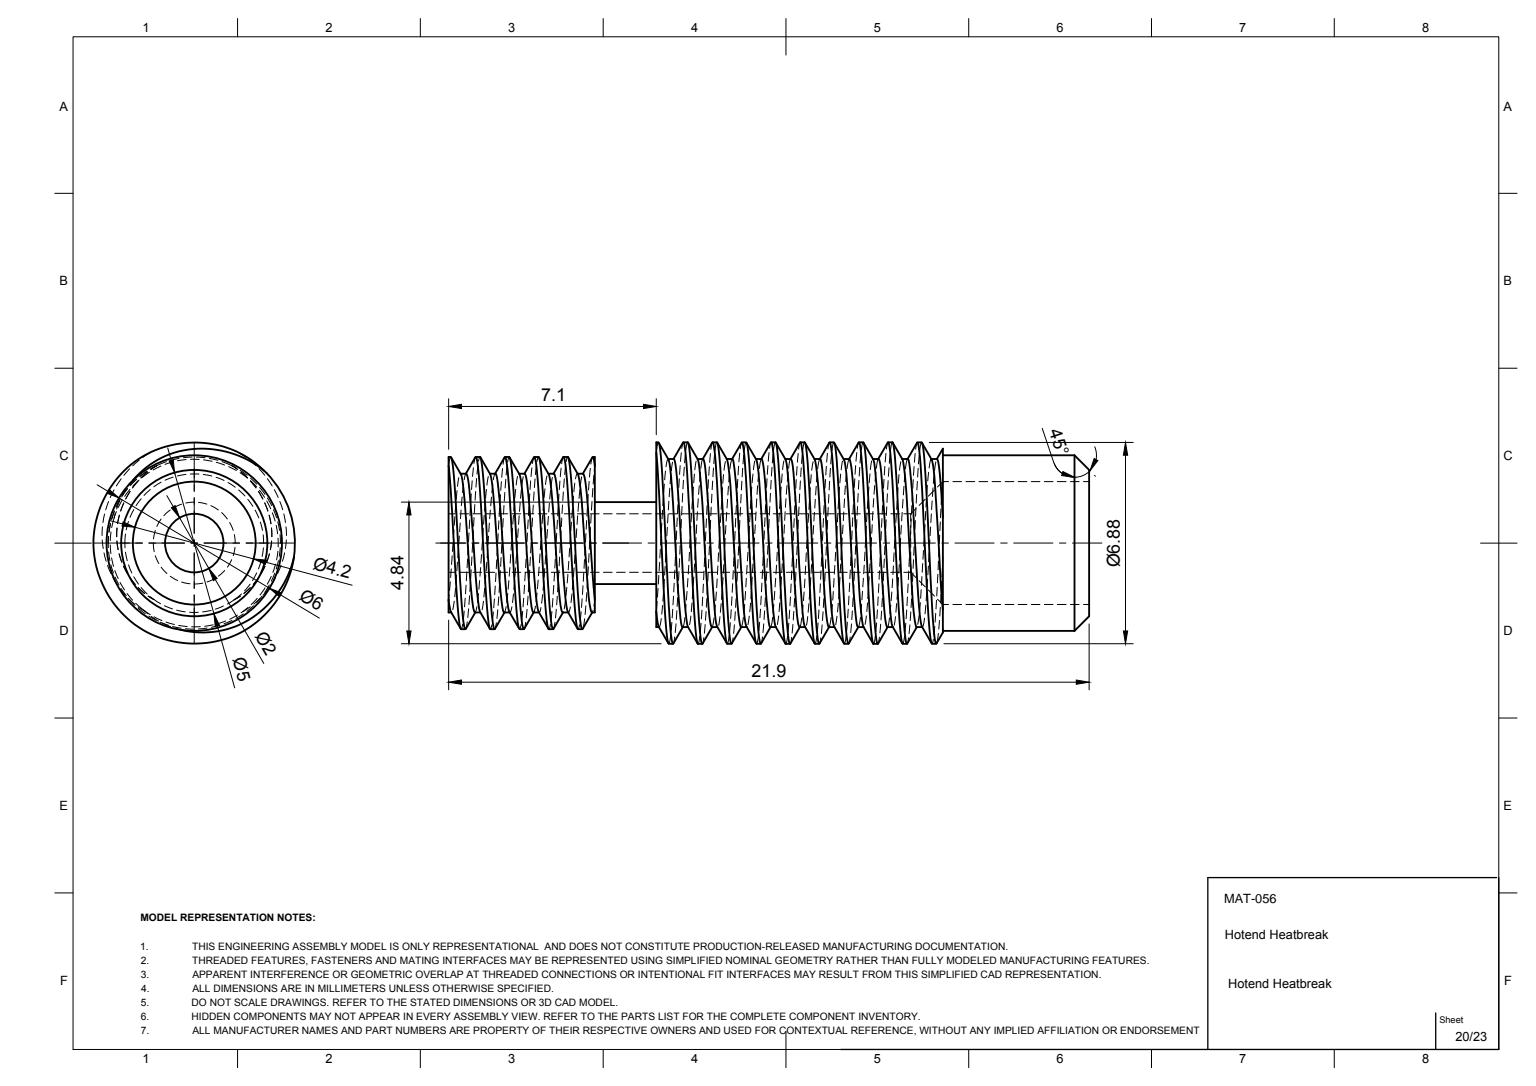
ISO-10303-21;
HEADER;
/* Generated by software containing ST-Developer
 * from STEP Tools, Inc. (www.steptools.com) 
 */

FILE_DESCRIPTION(
/* description */ (''),
/* implementation_level */ '2;1');

FILE_NAME(
/* name */ 'Hotend Heatbreak.step',
/* time_stamp */ '2026-10-28T16:47:13+01:00',
/* author */ (''),
/* organization */ (''),
/* preprocessor_version */ 'ST-DEVELOPER v20.2',
/* originating_system */ 'Autodesk Translation Framework v15.17.0.0',
/* authorisation */ '');

FILE_SCHEMA (('AUTOMOTIVE_DESIGN { 1 0 10303 214 3 1 1 }'));
ENDSEC;

DATA;
#10=MECHANICAL_DESIGN_GEOMETRIC_PRESENTATION_REPRESENTATION('',(#4610),#459242);
#4422=SHAPE_REPRESENTATION_RELATIONSHIP('SRR','None',#459349,#4443);
#4443=ADVANCED_BREP_SHAPE_REPRESENTATION('',(#4490),#459238);
#4490=MANIFOLD_SOLID_BREP('E3D V6 throat',#94668);
#4610=STYLED_ITEM('',(#459519),#4490);
#5107=CONICAL_SURFACE('',#105410,2.5,0.78539816339745);
#5108=CONICAL_SURFACE('',#105423,2.1,0.78539816339745);
#5260=FACE_BOUND('',#18019,.T.);
#5261=FACE_BOUND('',#18033,.T.);
#5262=FACE_BOUND('',#18036,.T.);
#5263=FACE_BOUND('',#18038,.T.);
#6128=PLANE('',#105401);
#6129=PLANE('',#105405);
#6130=PLANE('',#105427);
#6131=PLANE('',#105428);
#6132=PLANE('',#105429);
#6133=PLANE('',#105430);
#6345=B_SPLINE_SURFACE_WITH_KNOTS('',3,3,((#456005,#456006,#456007,#456008,
#456009,#456010,#456011,#456012,#456013,#456014,#456015,#456016,#456017,
#456018,#456019,#456020,#456021,#456022,#456023,#456024,#456025,#456026,
#456027,#456028,#456029,#456030,#456031,#456032,#456033,#456034,#456035,
#456036,#456037,#456038,#456039,#456040,#456041),(#456042,#456043,#456044,
#456045,#456046,#456047,#456048,#456049,#456050,#456051,#456052,#456053,
#456054,#456055,#456056,#456057,#456058,#456059,#456060,#456061,#456062,
#456063,#456064,#456065,#456066,#456067,#456068,#456069,#456070,#456071,
#456072,#456073,#456074,#456075,#456076,#456077,#456078),(#456079,#456080,
#456081,#456082,#456083,#456084,#456085,#456086,#456087,#456088,#456089,
#456090,#456091,#456092,#456093,#456094,#456095,#456096,#456097,#456098,
#456099,#456100,#456101,#456102,#456103,#456104,#456105,#456106,#456107,
#456108,#456109,#456110,#456111,#456112,#456113,#456114,#456115),(#456116,
#456117,#456118,#456119,#456120,#456121,#456122,#456123,#456124,#456125,
#456126,#456127,#456128,#456129,#456130,#456131,#456132,#456133,#456134,
#456135,#456136,#456137,#456138,#456139,#456140,#456141,#456142,#456143,
#456144,#456145,#456146,#456147,#456148,#456149,#456150,#456151,#456152)),
 .UNSPECIFIED.,.F.,.F.,.F.,(4,4),(4,1,1,1,1,1,1,1,1,1,1,1,1,1,1,1,1,1,1,
1,1,1,1,1,1,1,1,1,1,1,1,1,1,1,4),(0.,0.0658467982010768),(8.3074775524011,
9.29231769095425,10.2771578295074,11.2619979680605,12.2468381066137,13.2316782451668,
14.21651838372,15.2013585222731,16.1861986608263,17.1710387993794,18.1558789379326,
19.1407190764857,20.1255592150389,21.110399353592,22.0952394921452,23.0800796306983,
24.0649197692515,25.0497599078046,26.0346000463578,27.0194401849109,28.0042803234641,
28.9891204620172,29.9739606005704,30.9588007391235,31.9436408776767,32.9284810162298,
33.913321154783,34.8981612933361,35.8830014318893,36.8678415704424,37.8526817089956,
38.8375218475487,39.8223619861019,40.807202124655,41.7920422632082),
 .UNSPECIFIED.);
#6346=B_SPLINE_SURFACE_WITH_KNOTS('',3,3,((#456376,#456377,#456378,#456379,
#456380,#456381,#456382,#456383,#456384,#456385,#456386,#456387,#456388,
#456389,#456390,#456391,#456392,#456393,#456394,#456395,#456396,#456397,
#456398,#456399,#456400,#456401,#456402,#456403,#456404,#456405,#456406,
#456407,#456408,#456409,#456410,#456411,#456412),(#456413,#456414,#456415,
#456416,#456417,#456418,#456419,#456420,#456421,#456422,#456423,#456424,
#456425,#456426,#456427,#456428,#456429,#456430,#456431,#456432,#456433,
#456434,#456435,#456436,#456437,#456438,#456439,#456440,#456441,#456442,
#456443,#456444,#456445,#456446,#456447,#456448,#456449),(#456450,#456451,
#456452,#456453,#456454,#456455,#456456,#456457,#456458,#456459,#456460,
#456461,#456462,#456463,#456464,#456465,#456466,#456467,#456468,#456469,
#456470,#456471,#456472,#456473,#456474,#456475,#456476,#456477,#456478,
#456479,#456480,#456481,#456482,#456483,#456484,#456485,#456486),(#456487,
#456488,#456489,#456490,#456491,#456492,#456493,#456494,#456495,#456496,
#456497,#456498,#456499,#456500,#456501,#456502,#456503,#456504,#456505,
#456506,#456507,#456508,#456509,#456510,#456511,#456512,#456513,#456514,
#456515,#456516,#456517,#456518,#456519,#456520,#456521,#456522,#456523)),
 .UNSPECIFIED.,.F.,.F.,.F.,(4,4),(4,1,1,1,1,1,1,1,1,1,1,1,1,1,1,1,1,1,1,
1,1,1,1,1,1,1,1,1,1,1,1,1,1,1,4),(0.,0.0658467982010768),(11.6150328478183,
12.5998729863715,13.5847131249246,14.5695532634778,15.5543934020309,16.5392335405841,
17.5240736791372,18.5089138176904,19.4937539562435,20.4785940947967,21.4634342333498,
22.448274371903,23.4331145104561,24.4179546490093,25.4027947875624,26.3876349261156,
27.3724750646687,28.3573152032219,29.342155341775,30.3269954803282,31.3118356188813,
32.2966757574344,33.2815158959876,34.2663560345407,35.2511961730939,36.236036311647,
37.2208764502002,38.2057165887533,39.1905567273065,40.1753968658596,41.1602370044128,
42.1450771429659,43.1299172815191,44.1147574200722,45.0995975586254),
 .UNSPECIFIED.);
#6347=B_SPLINE_SURFACE_WITH_KNOTS('',3,3,((#456775,#456776,#456777,#456778,
#456779,#456780,#456781,#456782,#456783,#456784,#456785,#456786,#456787,
#456788,#456789,#456790,#456791,#456792,#456793,#456794,#456795,#456796,
#456797,#456798,#456799,#456800,#456801,#456802,#456803,#456804,#456805,
#456806,#456807,#456808,#456809,#456810,#456811,#456812,#456813,#456814,
#456815,#456816,#456817,#456818,#456819,#456820,#456821,#456822,#456823,
#456824,#456825,#456826,#456827,#456828,#456829,#456830,#456831,#456832,
#456833,#456834,#456835,#456836,#456837,#456838,#456839,#456840,#456841),
(#456842,#456843,#456844,#456845,#456846,#456847,#456848,#456849,#456850,
#456851,#456852,#456853,#456854,#456855,#456856,#456857,#456858,#456859,
#456860,#456861,#456862,#456863,#456864,#456865,#456866,#456867,#456868,
#456869,#456870,#456871,#456872,#456873,#456874,#456875,#456876,#456877,
#456878,#456879,#456880,#456881,#456882,#456883,#456884,#456885,#456886,
#456887,#456888,#456889,#456890,#456891,#456892,#456893,#456894,#456895,
#456896,#456897,#456898,#456899,#456900,#456901,#456902,#456903,#456904,
#456905,#456906,#456907,#456908),(#456909,#456910,#456911,#456912,#456913,
#456914,#456915,#456916,#456917,#456918,#456919,#456920,#456921,#456922,
#456923,#456924,#456925,#456926,#456927,#456928,#456929,#456930,#456931,
#456932,#456933,#456934,#456935,#456936,#456937,#456938,#456939,#456940,
#456941,#456942,#456943,#456944,#456945,#456946,#456947,#456948,#456949,
#456950,#456951,#456952,#456953,#456954,#456955,#456956,#456957,#456958,
#456959,#456960,#456961,#456962,#456963,#456964,#456965,#456966,#456967,
#456968,#456969,#456970,#456971,#456972,#456973,#456974,#456975),(#456976,
#456977,#456978,#456979,#456980,#456981,#456982,#456983,#456984,#456985,
#456986,#456987,#456988,#456989,#456990,#456991,#456992,#456993,#456994,
#456995,#456996,#456997,#456998,#456999,#457000,#457001,#457002,#457003,
#457004,#457005,#457006,#457007,#457008,#457009,#457010,#457011,#457012,
#457013,#457014,#457015,#457016,#457017,#457018,#457019,#457020,#457021,
#457022,#457023,#457024,#457025,#457026,#457027,#457028,#457029,#457030,
#457031,#457032,#457033,#457034,#457035,#457036,#457037,#457038,#457039,
#457040,#457041,#457042)),.UNSPECIFIED.,.F.,.F.,.F.,(4,4),(4,1,1,1,1,1,
1,1,1,1,1,1,1,1,1,1,1,1,1,1,1,1,1,1,1,1,1,1,1,1,1,1,1,1,1,1,1,1,1,1,1,1,
1,1,1,1,1,1,1,1,1,1,1,1,1,1,1,1,1,1,1,1,1,1,4),(0.,0.0658179306876173),
(8.30838445208317,9.30280550342046,10.2972265547578,11.2916476060951,12.2860686574324,
13.2804897087697,14.2749107601069,15.2693318114442,16.2637528627815,17.2581739141188,
18.2525949654561,19.2470160167934,20.2414370681307,21.235858119468,22.2302791708053,
23.2247002221426,24.2191212734799,25.2135423248172,26.2079633761545,27.2023844274918,
28.1968054788291,29.1912265301664,30.1856475815037,31.180068632841,32.1744896841783,
33.1689107355156,34.1633317868529,35.1577528381902,36.1521738895275,37.1465949408648,
38.1410159922021,39.1354370435394,40.1298580948767,41.1242791462139,42.1187001975512,
43.1131212488885,44.1075423002258,45.1019633515631,46.0963844029004,47.0908054542377,
48.085226505575,49.0796475569123,50.0740686082496,51.0684896595869,52.0629107109242,
53.0573317622615,54.0517528135988,55.0461738649361,56.0405949162734,57.0350159676107,
58.029437018948,59.0238580702853,60.0182791216226,61.0127001729599,62.0071212242972,
63.0015422756345,63.9959633269718,64.9903843783091,65.9848054296463,66.9792264809836,
67.9736475323209,68.9680685836582,69.9624896349955,70.9569106863328,71.9513317376701),
 .UNSPECIFIED.);
#6348=B_SPLINE_SURFACE_WITH_KNOTS('',3,3,((#457239,#457240,#457241,#457242,
#457243,#457244,#457245,#457246,#457247,#457248,#457249,#457250,#457251,
#457252,#457253,#457254,#457255,#457256,#457257,#457258,#457259,#457260,
#457261,#457262,#457263,#457264,#457265,#457266,#457267,#457268,#457269,
#457270,#457271,#457272,#457273,#457274,#457275,#457276,#457277,#457278,
#457279,#457280,#457281,#457282,#457283,#457284,#457285,#457286,#457287,
#457288,#457289,#457290,#457291,#457292,#457293,#457294,#457295,#457296,
#457297,#457298,#457299,#457300,#457301,#457302,#457303,#457304,#457305),
(#457306,#457307,#457308,#457309,#457310,#457311,#457312,#457313,#457314,
#457315,#457316,#457317,#457318,#457319,#457320,#457321,#457322,#457323,
#457324,#457325,#457326,#457327,#457328,#457329,#457330,#457331,#457332,
#457333,#457334,#457335,#457336,#457337,#457338,#457339,#457340,#457341,
#457342,#457343,#457344,#457345,#457346,#457347,#457348,#457349,#457350,
#457351,#457352,#457353,#457354,#457355,#457356,#457357,#457358,#457359,
#457360,#457361,#457362,#457363,#457364,#457365,#457366,#457367,#457368,
#457369,#457370,#457371,#457372),(#457373,#457374,#457375,#457376,#457377,
#457378,#457379,#457380,#457381,#457382,#457383,#457384,#457385,#457386,
#457387,#457388,#457389,#457390,#457391,#457392,#457393,#457394,#457395,
#457396,#457397,#457398,#457399,#457400,#457401,#457402,#457403,#457404,
#457405,#457406,#457407,#457408,#457409,#457410,#457411,#457412,#457413,
#457414,#457415,#457416,#457417,#457418,#457419,#457420,#457421,#457422,
#457423,#457424,#457425,#457426,#457427,#457428,#457429,#457430,#457431,
#457432,#457433,#457434,#457435,#457436,#457437,#457438,#457439),(#457440,
#457441,#457442,#457443,#457444,#457445,#457446,#457447,#457448,#457449,
#457450,#457451,#457452,#457453,#457454,#457455,#457456,#457457,#457458,
#457459,#457460,#457461,#457462,#457463,#457464,#457465,#457466,#457467,
#457468,#457469,#457470,#457471,#457472,#457473,#457474,#457475,#457476,
#457477,#457478,#457479,#457480,#457481,#457482,#457483,#457484,#457485,
#457486,#457487,#457488,#457489,#457490,#457491,#457492,#457493,#457494,
#457495,#457496,#457497,#457498,#457499,#457500,#457501,#457502,#457503,
#457504,#457505,#457506)),.UNSPECIFIED.,.F.,.F.,.F.,(4,4),(4,1,1,1,1,1,
1,1,1,1,1,1,1,1,1,1,1,1,1,1,1,1,1,1,1,1,1,1,1,1,1,1,1,1,1,1,1,1,1,1,1,1,
1,1,1,1,1,1,1,1,1,1,1,1,1,1,1,1,1,1,1,1,1,1,4),(0.,0.0658179306876173),
(11.6150328478183,12.6094538991556,13.6038749504929,14.5982960018302,15.5927170531675,
16.5871381045047,17.581559155842,18.5759802071793,19.5704012585166,20.5648223098539,
21.5592433611912,22.5536644125285,23.5480854638658,24.5425065152031,25.5369275665404,
26.5313486178777,27.525769669215,28.5201907205523,29.5146117718896,30.5090328232269,
31.5034538745642,32.4978749259015,33.4922959772388,34.4867170285761,35.4811380799134,
36.4755591312507,37.469980182588,38.4644012339253,39.4588222852626,40.4532433365999,
41.4476643879372,42.4420854392745,43.4365064906117,44.430927541949,45.4253485932863,
46.4197696446236,47.4141906959609,48.4086117472982,49.4030327986355,50.3974538499728,
51.3918749013101,52.3862959526474,53.3807170039847,54.375138055322,55.3695591066593,
56.3639801579966,57.3584012093339,58.3528222606712,59.3472433120085,60.3416643633458,
61.3360854146831,62.3305064660204,63.3249275173577,64.319348568695,65.3137696200323,
66.3081906713696,67.3026117227069,68.2970327740442,69.2914538253815,70.2858748767188,
71.280295928056,72.2747169793933,73.2691380307306,74.2635590820679,75.2579801334052),
 .UNSPECIFIED.);
#12030=FACE_OUTER_BOUND('',#17985,.T.);
#12031=FACE_OUTER_BOUND('',#17986,.T.);
#12032=FACE_OUTER_BOUND('',#17987,.T.);
#12033=FACE_OUTER_BOUND('',#17988,.T.);
#12034=FACE_OUTER_BOUND('',#17989,.T.);
#12035=FACE_OUTER_BOUND('',#17990,.T.);
#12036=FACE_OUTER_BOUND('',#17991,.T.);
#12037=FACE_OUTER_BOUND('',#17992,.T.);
#12038=FACE_OUTER_BOUND('',#17993,.T.);
#12039=FACE_OUTER_BOUND('',#17994,.T.);
#12040=FACE_OUTER_BOUND('',#17995,.T.);
#12041=FACE_OUTER_BOUND('',#17996,.T.);
#12042=FACE_OUTER_BOUND('',#17997,.T.);
#12043=FACE_OUTER_BOUND('',#17998,.T.);
#12044=FACE_OUTER_BOUND('',#17999,.T.);
#12045=FACE_OUTER_BOUND('',#18000,.T.);
#12046=FACE_OUTER_BOUND('',#18001,.T.);
#12047=FACE_OUTER_BOUND('',#18002,.T.);
#12048=FACE_OUTER_BOUND('',#18003,.T.);
#12049=FACE_OUTER_BOUND('',#18004,.T.);
#12050=FACE_OUTER_BOUND('',#18005,.T.);
#12051=FACE_OUTER_BOUND('',#18006,.T.);
#12052=FACE_OUTER_BOUND('',#18007,.T.);
#12053=FACE_OUTER_BOUND('',#18008,.T.);
#12054=FACE_OUTER_BOUND('',#18009,.T.);
#12055=FACE_OUTER_BOUND('',#18010,.T.);
#12056=FACE_OUTER_BOUND('',#18011,.T.);
#12057=FACE_OUTER_BOUND('',#18012,.T.);
#12058=FACE_OUTER_BOUND('',#18013,.T.);
#12059=FACE_OUTER_BOUND('',#18014,.T.);
#12060=FACE_OUTER_BOUND('',#18015,.T.);
#12061=FACE_OUTER_BOUND('',#18016,.T.);
#12062=FACE_OUTER_BOUND('',#18017,.T.);
#12063=FACE_OUTER_BOUND('',#18018,.T.);
#12064=FACE_OUTER_BOUND('',#18020,.T.);
#12065=FACE_OUTER_BOUND('',#18021,.T.);
#12066=FACE_OUTER_BOUND('',#18022,.T.);
#12067=FACE_OUTER_BOUND('',#18023,.T.);
#12068=FACE_OUTER_BOUND('',#18024,.T.);
#12069=FACE_OUTER_BOUND('',#18025,.T.);
#12070=FACE_OUTER_BOUND('',#18026,.T.);
#12071=FACE_OUTER_BOUND('',#18027,.T.);
#12072=FACE_OUTER_BOUND('',#18028,.T.);
#12073=FACE_OUTER_BOUND('',#18029,.T.);
#12074=FACE_OUTER_BOUND('',#18030,.T.);
#12075=FACE_OUTER_BOUND('',#18031,.T.);
#12076=FACE_OUTER_BOUND('',#18032,.T.);
#12077=FACE_OUTER_BOUND('',#18034,.T.);
#12078=FACE_OUTER_BOUND('',#18035,.T.);
#12079=FACE_OUTER_BOUND('',#18037,.T.);
#17985=EDGE_LOOP('',(#86428,#86429,#86430,#86431));
#17986=EDGE_LOOP('',(#86432,#86433,#86434,#86435));
#17987=EDGE_LOOP('',(#86436,#86437,#86438,#86439));
#17988=EDGE_LOOP('',(#86440,#86441,#86442,#86443));
#17989=EDGE_LOOP('',(#86444,#86445,#86446,#86447));
#17990=EDGE_LOOP('',(#86448,#86449,#86450,#86451));
#17991=EDGE_LOOP('',(#86452,#86453,#86454,#86455));
#17992=EDGE_LOOP('',(#86456,#86457,#86458,#86459));
#17993=EDGE_LOOP('',(#86460,#86461,#86462,#86463));
#17994=EDGE_LOOP('',(#86464,#86465,#86466,#86467));
#17995=EDGE_LOOP('',(#86468,#86469,#86470));
#17996=EDGE_LOOP('',(#86471,#86472,#86473,#86474,#86475));
#17997=EDGE_LOOP('',(#86476,#86477,#86478,#86479));
#17998=EDGE_LOOP('',(#86480,#86481,#86482,#86483));
#17999=EDGE_LOOP('',(#86484,#86485,#86486,#86487));
#18000=EDGE_LOOP('',(#86488,#86489,#86490,#86491));
#18001=EDGE_LOOP('',(#86492,#86493,#86494,#86495));
#18002=EDGE_LOOP('',(#86496,#86497,#86498,#86499));
#18003=EDGE_LOOP('',(#86500,#86501,#86502,#86503));
#18004=EDGE_LOOP('',(#86504,#86505,#86506,#86507));
#18005=EDGE_LOOP('',(#86508,#86509,#86510,#86511));
#18006=EDGE_LOOP('',(#86512,#86513,#86514,#86515));
#18007=EDGE_LOOP('',(#86516,#86517,#86518,#86519));
#18008=EDGE_LOOP('',(#86520,#86521,#86522,#86523));
#18009=EDGE_LOOP('',(#86524,#86525,#86526,#86527));
#18010=EDGE_LOOP('',(#86528,#86529,#86530,#86531));
#18011=EDGE_LOOP('',(#86532,#86533,#86534,#86535));
#18012=EDGE_LOOP('',(#86536,#86537,#86538,#86539));
#18013=EDGE_LOOP('',(#86540,#86541,#86542,#86543));
#18014=EDGE_LOOP('',(#86544,#86545,#86546,#86547));
#18015=EDGE_LOOP('',(#86548,#86549,#86550,#86551,#86552,#86553,#86554,#86555,
#86556,#86557,#86558,#86559,#86560,#86561));
#18016=EDGE_LOOP('',(#86562,#86563,#86564,#86565));
#18017=EDGE_LOOP('',(#86566,#86567,#86568,#86569,#86570,#86571,#86572,#86573,
#86574,#86575,#86576,#86577,#86578,#86579));
#18018=EDGE_LOOP('',(#86580,#86581,#86582,#86583));
#18019=EDGE_LOOP('',(#86584));
#18020=EDGE_LOOP('',(#86585,#86586,#86587,#86588));
#18021=EDGE_LOOP('',(#86589,#86590,#86591,#86592,#86593,#86594));
#18022=EDGE_LOOP('',(#86595,#86596,#86597,#86598,#86599,#86600,#86601,#86602,
#86603,#86604,#86605,#86606,#86607,#86608,#86609,#86610,#86611,#86612,#86613,
#86614,#86615,#86616,#86617,#86618));
#18023=EDGE_LOOP('',(#86619,#86620,#86621,#86622));
#18024=EDGE_LOOP('',(#86623,#86624,#86625,#86626,#86627,#86628,#86629,#86630,
#86631,#86632,#86633,#86634,#86635,#86636,#86637,#86638,#86639,#86640,#86641,
#86642,#86643,#86644,#86645,#86646,#86647));
#18025=EDGE_LOOP('',(#86648,#86649,#86650,#86651,#86652));
#18026=EDGE_LOOP('',(#86653,#86654,#86655,#86656));
#18027=EDGE_LOOP('',(#86657,#86658,#86659,#86660));
#18028=EDGE_LOOP('',(#86661,#86662,#86663,#86664,#86665,#86666,#86667));
#18029=EDGE_LOOP('',(#86668,#86669,#86670,#86671));
#18030=EDGE_LOOP('',(#86672,#86673,#86674,#86675));
#18031=EDGE_LOOP('',(#86676,#86677,#86678,#86679));
#18032=EDGE_LOOP('',(#86680));
#18033=EDGE_LOOP('',(#86681));
#18034=EDGE_LOOP('',(#86682,#86683,#86684,#86685));
#18035=EDGE_LOOP('',(#86686,#86687,#86688,#86689));
#18036=EDGE_LOOP('',(#86690));
#18037=EDGE_LOOP('',(#86691,#86692,#86693,#86694));
#18038=EDGE_LOOP('',(#86695));
#23442=CIRCLE('',#105365,3.442);
#23443=CIRCLE('',#105376,2.872);
#23444=CIRCLE('',#105378,2.872);
#23445=CIRCLE('',#105388,2.942);
#23446=CIRCLE('',#105394,2.37175);
#23447=CIRCLE('',#105400,2.37175);
#23448=CIRCLE('',#105402,2.942);
#23449=CIRCLE('',#105403,1.4);
#23450=CIRCLE('',#105406,3.);
#23451=CIRCLE('',#105407,3.);
#23452=CIRCLE('',#105409,2.872);
#23453=CIRCLE('',#105411,3.);
#23454=CIRCLE('',#105412,3.);
#23455=CIRCLE('',#105413,2.5);
#23456=CIRCLE('',#105415,1.4);
#23457=CIRCLE('',#105417,3.442);
#23458=CIRCLE('',#105419,3.);
#23459=CIRCLE('',#105421,2.1);
#23460=CIRCLE('',#105422,2.1);
#23461=CIRCLE('',#105424,1.);
#23462=CIRCLE('',#105426,1.);
#26936=B_SPLINE_CURVE_WITH_KNOTS('',3,(#454971,#454972,#454973,#454974,
#454975,#454976,#454977,#454978,#454979,#454980),.UNSPECIFIED.,.F.,.F.,
(4,3,3,4),(-4.09293042013066,-3.97768420534918,-2.98326315401189,-2.06773127522702),
 .UNSPECIFIED.);
#26937=B_SPLINE_CURVE_WITH_KNOTS('',3,(#454983,#454984,#454985,#454986,
#454987,#454988,#454989),.UNSPECIFIED.,.F.,.F.,(4,3,4),(0.,0.994421051337293,
1.11639350868612),.UNSPECIFIED.);
#26938=B_SPLINE_CURVE_WITH_KNOTS('',3,(#454994,#454995,#454996,#454997,
#454998,#454999,#455000,#455001,#455002,#455003,#455004,#455005,#455006,
#455007,#455008,#455009,#455010,#455011,#455012,#455013,#455014,#455015),
 .UNSPECIFIED.,.F.,.F.,(4,3,3,3,3,3,3,4),(-10.3761157273102,-9.94421051337296,
-8.94978946203567,-7.95536841069837,-6.96094735936108,-5.96652630802378,
-4.97210525668648,-4.09293042013066),.UNSPECIFIED.);
#26939=B_SPLINE_CURVE_WITH_KNOTS('',3,(#455016,#455017,#455018,#455019,
#455020,#455021,#455022,#455023,#455024,#455025,#455026,#455027,#455028,
#455029,#455030,#455031,#455032,#455033,#455034,#455035,#455036,#455037),
 .UNSPECIFIED.,.F.,.F.,(4,3,3,3,3,3,3,4),(1.11639350868612,1.98884210267459,
2.98326315401189,3.97768420534918,4.97210525668648,5.96652630802378,6.96094735936107,
7.39957881586571),.UNSPECIFIED.);
#26940=B_SPLINE_CURVE_WITH_KNOTS('',3,(#455042,#455043,#455044,#455045,
#455046,#455047,#455048,#455049,#455050,#455051,#455052,#455053,#455054,
#455055,#455056,#455057,#455058,#455059,#455060,#455061,#455062,#455063),
 .UNSPECIFIED.,.F.,.F.,(4,3,3,3,3,3,3,4),(-16.6593010344898,-15.9107368213967,
-14.9163157700594,-13.9218947187222,-12.9274736673849,-11.9330526160476,
-10.9386315647103,-10.3761157273102),.UNSPECIFIED.);
#26941=B_SPLINE_CURVE_WITH_KNOTS('',3,(#455064,#455065,#455066,#455067,
#455068,#455069,#455070,#455071,#455072,#455073,#455074,#455075,#455076,
#455077,#455078,#455079,#455080,#455081,#455082,#455083,#455084,#455085),
 .UNSPECIFIED.,.F.,.F.,(4,3,3,3,3,3,3,4),(7.39957881586571,7.95536841069837,
8.94978946203567,9.94421051337297,10.9386315647103,11.9330526160476,12.9274736673849,
13.6827641230453),.UNSPECIFIED.);
#26942=B_SPLINE_CURVE_WITH_KNOTS('',3,(#455090,#455091,#455092,#455093,
#455094,#455095,#455096,#455097,#455098,#455099,#455100,#455101,#455102,
#455103,#455104,#455105,#455106,#455107,#455108,#455109,#455110,#455111,
#455112,#455113,#455114),.UNSPECIFIED.,.F.,.F.,(4,3,3,3,3,3,3,3,4),(-22.9424863416694,
-22.8716841807578,-21.8772631294205,-20.8828420780832,-19.8884210267459,
-18.8939999754086,-17.8995789240713,-16.905157872734,-16.6593010344898),
 .UNSPECIFIED.);
#26943=B_SPLINE_CURVE_WITH_KNOTS('',3,(#455115,#455116,#455117,#455118,
#455119,#455120,#455121,#455122,#455123,#455124,#455125,#455126,#455127,
#455128,#455129,#455130,#455131,#455132,#455133,#455134,#455135,#455136,
#455137,#455138,#455139),.UNSPECIFIED.,.F.,.F.,(4,3,3,3,3,3,3,3,4),(13.6827641230453,
13.9218947187222,14.9163157700594,15.9107368213967,16.905157872734,17.8995789240713,
18.8939999754086,19.8884210267459,19.9659494302249),.UNSPECIFIED.);
#26944=B_SPLINE_CURVE_WITH_KNOTS('',3,(#455144,#455145,#455146,#455147,
#455148,#455149,#455150,#455151,#455152,#455153,#455154,#455155,#455156,
#455157,#455158,#455159,#455160,#455161,#455162,#455163,#455164,#455165),
 .UNSPECIFIED.,.F.,.F.,(4,3,3,3,3,3,3,4),(-29.225671648849,-28.8382104887816,
-27.8437894374443,-26.849368386107,-25.8549473347697,-24.8605262834324,
-23.8661052320951,-22.9424863416694),.UNSPECIFIED.);
#26945=B_SPLINE_CURVE_WITH_KNOTS('',3,(#455166,#455167,#455168,#455169,
#455170,#455171,#455172,#455173,#455174,#455175,#455176,#455177,#455178,
#455179,#455180,#455181,#455182,#455183,#455184,#455185,#455186,#455187),
 .UNSPECIFIED.,.F.,.F.,(4,3,3,3,3,3,3,4),(19.9659494302249,20.8828420780832,
21.8772631294205,22.8716841807578,23.8661052320951,24.8605262834324,25.8549473347697,
26.2491347374045),.UNSPECIFIED.);
#26946=B_SPLINE_CURVE_WITH_KNOTS('',3,(#455192,#455193,#455194,#455195,
#455196,#455197,#455198,#455199,#455200,#455201,#455202,#455203,#455204,
#455205,#455206,#455207,#455208,#455209,#455210,#455211,#455212,#455213),
 .UNSPECIFIED.,.F.,.F.,(4,3,3,3,3,3,3,4),(-35.5088569560286,-34.8047367968054,
-33.8103157454681,-32.8158946941308,-31.8214736427935,-30.8270525914562,
-29.8326315401189,-29.225671648849),.UNSPECIFIED.);
#26947=B_SPLINE_CURVE_WITH_KNOTS('',3,(#455214,#455215,#455216,#455217,
#455218,#455219,#455220,#455221,#455222,#455223,#455224,#455225,#455226,
#455227,#455228,#455229,#455230,#455231,#455232,#455233,#455234,#455235),
 .UNSPECIFIED.,.F.,.F.,(4,3,3,3,3,3,3,4),(26.2491347374045,26.849368386107,
27.8437894374443,28.8382104887816,29.8326315401189,30.8270525914562,31.8214736427935,
32.532320044584),.UNSPECIFIED.);
#26948=B_SPLINE_CURVE_WITH_KNOTS('',3,(#455240,#455241,#455242,#455243,
#455244,#455245,#455246,#455247,#455248,#455249,#455250,#455251,#455252,
#455253,#455254,#455255,#455256,#455257,#455258,#455259,#455260,#455261,
#455262,#455263,#455264),.UNSPECIFIED.,.F.,.F.,(4,3,3,3,3,3,3,3,4),(-41.7920422632082,
-41.7656841561665,-40.7712631048292,-39.7768420534919,-38.7824210021546,
-37.7879999508173,-36.79357889948,-35.7991578481427,-35.5088569560286),
 .UNSPECIFIED.);
#26949=B_SPLINE_CURVE_WITH_KNOTS('',3,(#455265,#455266,#455267,#455268,
#455269,#455270,#455271,#455272,#455273,#455274,#455275,#455276,#455277,
#455278,#455279,#455280,#455281,#455282,#455283,#455284,#455285,#455286,
#455287,#455288,#455289),.UNSPECIFIED.,.F.,.F.,(4,3,3,3,3,3,3,3,4),(32.532320044584,
32.8158946941308,33.8103157454681,34.8047367968054,35.7991578481427,36.79357889948,
37.7879999508173,38.7824210021546,38.8155053517636),.UNSPECIFIED.);
#26950=B_SPLINE_CURVE_WITH_KNOTS('',3,(#455294,#455295,#455296,#455297,
#455298,#455299,#455300,#455301,#455302,#455303,#455304,#455305,#455306,
#455307,#455308,#455309,#455310,#455311,#455312,#455313,#455314,#455315),
 .UNSPECIFIED.,.F.,.F.,(4,3,3,3,3,3,3,4),(-48.0752275703878,-47.7322104641902,
-46.7377894128529,-45.7433683615156,-44.7489473101783,-43.754526258841,
-42.7601052075037,-41.7920422632082),.UNSPECIFIED.);
#26951=B_SPLINE_CURVE_WITH_KNOTS('',3,(#455316,#455317,#455318,#455319,
#455320,#455321,#455322,#455323,#455324,#455325,#455326,#455327,#455328,
#455329,#455330,#455331,#455332,#455333,#455334,#455335,#455336,#455337),
 .UNSPECIFIED.,.F.,.F.,(4,3,3,3,3,3,3,4),(38.8155053517636,39.7768420534919,
40.7712631048292,41.7656841561664,42.7601052075037,43.754526258841,44.7489473101783,
45.0986906589432),.UNSPECIFIED.);
#26952=B_SPLINE_CURVE_WITH_KNOTS('',3,(#455342,#455343,#455344,#455345,
#455346,#455347,#455348,#455349,#455350,#455351,#455352,#455353,#455354,
#455355,#455356,#455357,#455358,#455359,#455360,#455361,#455362,#455363),
 .UNSPECIFIED.,.F.,.F.,(4,3,3,3,3,3,3,4),(-54.3584128775674,-53.698736772214,
-52.7043157208767,-51.7098946695394,-50.7154736182021,-49.7210525668648,
-48.7266315155275,-48.0752275703878),.UNSPECIFIED.);
#26953=B_SPLINE_CURVE_WITH_KNOTS('',3,(#455364,#455365,#455366,#455367,
#455368,#455369,#455370,#455371,#455372,#455373,#455374,#455375,#455376,
#455377,#455378,#455379,#455380,#455381,#455382,#455383,#455384,#455385),
 .UNSPECIFIED.,.F.,.F.,(4,3,3,3,3,3,3,4),(45.0986906589432,45.7433683615156,
46.7377894128529,47.7322104641902,48.7266315155275,49.7210525668648,50.7154736182021,
51.3818759661228),.UNSPECIFIED.);
#26954=B_SPLINE_CURVE_WITH_KNOTS('',3,(#455390,#455391,#455392,#455393,
#455394,#455395,#455396,#455397,#455398,#455399,#455400,#455401,#455402,
#455403,#455404,#455405,#455406,#455407,#455408,#455409,#455410,#455411),
 .UNSPECIFIED.,.F.,.F.,(4,3,3,3,3,3,3,4),(-60.641598184747,-59.6652630802378,
-58.6708420289005,-57.6764209775632,-56.6819999262259,-55.6875788748886,
-54.6931578235513,-54.3584128775674),.UNSPECIFIED.);
#26955=B_SPLINE_CURVE_WITH_KNOTS('',3,(#455412,#455413,#455414,#455415,
#455416,#455417,#455418,#455419,#455420,#455421,#455422,#455423,#455424,
#455425,#455426,#455427,#455428,#455429,#455430,#455431,#455432,#455433),
 .UNSPECIFIED.,.F.,.F.,(4,3,3,3,3,3,3,4),(51.3818759661228,51.7098946695394,
52.7043157208767,53.698736772214,54.6931578235513,55.6875788748886,56.6819999262259,
57.6650612733024),.UNSPECIFIED.);
#26956=B_SPLINE_CURVE_WITH_KNOTS('',3,(#455439,#455440,#455441,#455442,
#455443),.UNSPECIFIED.,.F.,.F.,(4,1,4),(72.2566310325653,72.2747169793933,
73.1902488581782),.UNSPECIFIED.);
#26957=B_SPLINE_CURVE_WITH_KNOTS('',3,(#455449,#455450,#455451,#455452,
#455453,#455454,#455455,#455456,#455457,#455458),.UNSPECIFIED.,.F.,.F.,
(4,1,1,1,1,1,1,4),(65.9734457253856,66.3081906713696,67.3026117227069,68.2970327740442,
69.2914538253815,70.2858748767188,71.280295928056,72.2566310325653),
 .UNSPECIFIED.);
#26958=B_SPLINE_CURVE_WITH_KNOTS('',3,(#455461,#455462,#455463,#455464,
#455465,#455466,#455467,#455468,#455469,#455470),.UNSPECIFIED.,.F.,.F.,
(4,1,1,1,1,1,1,4),(65.9734457253856,65.9848054296463,66.9792264809836,67.9736475323209,
68.9680685836582,69.9624896349955,70.9569106863328,71.9513317376701),
 .UNSPECIFIED.);
#26959=B_SPLINE_CURVE_WITH_KNOTS('',3,(#455475,#455476,#455477,#455478,
#455479,#455480,#455481,#455482,#455483,#455484),.UNSPECIFIED.,.F.,.F.,
(4,1,1,1,1,1,1,4),(59.6902604182061,60.3416643633458,61.3360854146831,62.3305064660204,
63.3249275173577,64.319348568695,65.3137696200323,65.9734457253856),
 .UNSPECIFIED.);
#26960=B_SPLINE_CURVE_WITH_KNOTS('',3,(#455485,#455486,#455487,#455488,
#455489,#455490,#455491,#455492,#455493,#455494),.UNSPECIFIED.,.F.,.F.,
(4,1,1,1,1,1,1,4),(59.6902604182061,60.0182791216226,61.0127001729599,62.0071212242972,
63.0015422756345,63.9959633269718,64.9903843783091,65.9734457253856),
 .UNSPECIFIED.);
#26961=B_SPLINE_CURVE_WITH_KNOTS('',3,(#455499,#455500,#455501,#455502,
#455503,#455504,#455505,#455506,#455507,#455508),.UNSPECIFIED.,.F.,.F.,
(4,1,1,1,1,1,1,4),(53.4070751110265,54.375138055322,55.3695591066593,56.3639801579966,
57.3584012093339,58.3528222606712,59.3472433120085,59.6902604182061),
 .UNSPECIFIED.);
#26962=B_SPLINE_CURVE_WITH_KNOTS('',3,(#455509,#455510,#455511,#455512,
#455513,#455514,#455515,#455516,#455517,#455518),.UNSPECIFIED.,.F.,.F.,
(4,1,1,1,1,1,1,4),(53.4070751110265,54.0517528135988,55.0461738649361,56.0405949162734,
57.0350159676107,58.029437018948,59.0238580702853,59.6902604182061),
 .UNSPECIFIED.);
#26963=B_SPLINE_CURVE_WITH_KNOTS('',3,(#455523,#455524,#455525,#455526,
#455527,#455528,#455529,#455530,#455531,#455532,#455533),.UNSPECIFIED.,
 .F.,.F.,(4,1,1,1,1,1,1,1,4),(47.1238898038469,47.4141906959609,48.4086117472982,
49.4030327986355,50.3974538499728,51.3918749013101,52.3862959526474,53.3807170039847,
53.4070751110265),.UNSPECIFIED.);
#26964=B_SPLINE_CURVE_WITH_KNOTS('',3,(#455534,#455535,#455536,#455537,
#455538,#455539,#455540,#455541,#455542,#455543),.UNSPECIFIED.,.F.,.F.,
(4,1,1,1,1,1,1,4),(47.1238898038469,48.085226505575,49.0796475569123,50.0740686082496,
51.0684896595869,52.0629107109242,53.0573317622615,53.4070751110265),
 .UNSPECIFIED.);
#26965=B_SPLINE_CURVE_WITH_KNOTS('',3,(#455548,#455549,#455550,#455551,
#455552,#455553,#455554,#455555,#455556,#455557),.UNSPECIFIED.,.F.,.F.,
(4,1,1,1,1,1,1,4),(40.8407044966673,41.4476643879372,42.4420854392745,43.4365064906117,
44.430927541949,45.4253485932863,46.4197696446236,47.1238898038469),
 .UNSPECIFIED.);
#26966=B_SPLINE_CURVE_WITH_KNOTS('',3,(#455558,#455559,#455560,#455561,
#455562,#455563,#455564,#455565,#455566,#455567,#455568),.UNSPECIFIED.,
 .F.,.F.,(4,1,1,1,1,1,1,1,4),(40.8407044966673,41.1242791462139,42.1187001975512,
43.1131212488885,44.1075423002258,45.1019633515631,46.0963844029004,47.0908054542377,
47.1238898038469),.UNSPECIFIED.);
#26967=B_SPLINE_CURVE_WITH_KNOTS('',3,(#455573,#455574,#455575,#455576,
#455577,#455578,#455579,#455580,#455581,#455582),.UNSPECIFIED.,.F.,.F.,
(4,1,1,1,1,1,1,4),(34.5575191894877,35.4811380799134,36.4755591312507,37.469980182588,
38.4644012339253,39.4588222852626,40.4532433365999,40.8407044966673),
 .UNSPECIFIED.);
#26968=B_SPLINE_CURVE_WITH_KNOTS('',3,(#455583,#455584,#455585,#455586,
#455587,#455588,#455589,#455590,#455591,#455592),.UNSPECIFIED.,.F.,.F.,
(4,1,1,1,1,1,1,4),(34.5575191894877,35.1577528381902,36.1521738895275,37.1465949408648,
38.1410159922021,39.1354370435394,40.1298580948767,40.8407044966673),
 .UNSPECIFIED.);
#26969=B_SPLINE_CURVE_WITH_KNOTS('',3,(#455597,#455598,#455599,#455600,
#455601,#455602,#455603,#455604,#455605,#455606,#455607),.UNSPECIFIED.,
 .F.,.F.,(4,1,1,1,1,1,1,1,4),(28.2743338823081,28.5201907205523,29.5146117718896,
30.5090328232269,31.5034538745642,32.4978749259015,33.4922959772388,34.4867170285761,
34.5575191894877),.UNSPECIFIED.);
#26970=B_SPLINE_CURVE_WITH_KNOTS('',3,(#455608,#455609,#455610,#455611,
#455612,#455613,#455614,#455615,#455616,#455617),.UNSPECIFIED.,.F.,.F.,
(4,1,1,1,1,1,1,4),(28.2743338823081,29.1912265301664,30.1856475815037,31.180068632841,
32.1744896841783,33.1689107355156,34.1633317868529,34.5575191894877),
 .UNSPECIFIED.);
#26971=B_SPLINE_CURVE_WITH_KNOTS('',3,(#455622,#455623,#455624,#455625,
#455626,#455627,#455628,#455629,#455630,#455631),.UNSPECIFIED.,.F.,.F.,
(4,1,1,1,1,1,1,4),(21.9911485751285,22.5536644125285,23.5480854638658,24.5425065152031,
25.5369275665404,26.5313486178777,27.525769669215,28.2743338823081),
 .UNSPECIFIED.);
#26972=B_SPLINE_CURVE_WITH_KNOTS('',3,(#455632,#455633,#455634,#455635,
#455636,#455637,#455638,#455639,#455640,#455641,#455642),.UNSPECIFIED.,
 .F.,.F.,(4,1,1,1,1,1,1,1,4),(21.9911485751285,22.2302791708053,23.2247002221426,
24.2191212734799,25.2135423248172,26.2079633761545,27.2023844274918,28.1968054788291,
28.2743338823081),.UNSPECIFIED.);
#26973=B_SPLINE_CURVE_WITH_KNOTS('',3,(#455647,#455648,#455649,#455650,
#455651,#455652,#455653,#455654,#455655,#455656),.UNSPECIFIED.,.F.,.F.,
(4,1,1,1,1,1,1,4),(15.7079632679489,16.5871381045047,17.581559155842,18.5759802071793,
19.5704012585166,20.5648223098539,21.5592433611912,21.9911485751285),
 .UNSPECIFIED.);
#26974=B_SPLINE_CURVE_WITH_KNOTS('',3,(#455657,#455658,#455659,#455660,
#455661,#455662,#455663,#455664,#455665,#455666),.UNSPECIFIED.,.F.,.F.,
(4,1,1,1,1,1,1,4),(15.7079632679489,16.2637528627815,17.2581739141188,18.2525949654561,
19.2470160167934,20.2414370681307,21.235858119468,21.9911485751285),
 .UNSPECIFIED.);
#26975=B_SPLINE_CURVE_WITH_KNOTS('',3,(#455672,#455673,#455674,#455675,
#455676,#455677,#455678,#455679,#455680,#455681),.UNSPECIFIED.,.F.,.F.,
(4,3,3,4),(-4.09293042013064,-3.9393605542126,-2.95452041565945,-2.06863817490912),
 .UNSPECIFIED.);
#26976=B_SPLINE_CURVE_WITH_KNOTS('',3,(#455684,#455685,#455686,#455687,
#455688,#455689,#455690),.UNSPECIFIED.,.F.,.F.,(4,3,4),(0.,0.984840138553148,
1.11730040836828),.UNSPECIFIED.);
#26977=B_SPLINE_CURVE_WITH_KNOTS('',3,(#455695,#455696,#455697,#455698,
#455699,#455700,#455701,#455702,#455703,#455704,#455705,#455706,#455707,
#455708,#455709,#455710,#455711,#455712,#455713,#455714,#455715,#455716),
 .UNSPECIFIED.,.F.,.F.,(4,3,3,3,3,3,3,4),(-10.3761157273102,-9.84840138553149,
-8.86356124697834,-7.87872110842519,-6.89388096987204,-5.9090408313189,
-4.92420069276575,-4.09293042013064),.UNSPECIFIED.);
#26978=B_SPLINE_CURVE_WITH_KNOTS('',3,(#455717,#455718,#455719,#455720,
#455721,#455722,#455723,#455724,#455725,#455726,#455727,#455728,#455729,
#455730,#455731,#455732,#455733,#455734,#455735,#455736,#455737,#455738),
 .UNSPECIFIED.,.F.,.F.,(4,3,3,3,3,3,3,4),(1.11730040836828,1.9696802771063,
2.95452041565944,3.93936055421259,4.92420069276574,5.90904083131889,6.89388096987204,
7.40048571554787),.UNSPECIFIED.);
#26979=B_SPLINE_CURVE_WITH_KNOTS('',3,(#455743,#455744,#455745,#455746,
#455747,#455748,#455749,#455750,#455751,#455752,#455753,#455754,#455755,
#455756,#455757,#455758,#455759,#455760,#455761,#455762,#455763,#455764),
 .UNSPECIFIED.,.F.,.F.,(4,3,3,3,3,3,3,4),(-16.6593010344898,-15.7574422168504,
-14.7726020782972,-13.7877619397441,-12.8029218011909,-11.8180816626378,
-10.8332415240846,-10.3761157273102),.UNSPECIFIED.);
#26980=B_SPLINE_CURVE_WITH_KNOTS('',3,(#455765,#455766,#455767,#455768,
#455769,#455770,#455771,#455772,#455773,#455774,#455775,#455776,#455777,
#455778,#455779,#455780,#455781,#455782,#455783,#455784,#455785,#455786),
 .UNSPECIFIED.,.F.,.F.,(4,3,3,3,3,3,3,4),(7.40048571554787,7.87872110842519,
8.86356124697834,9.84840138553149,10.8332415240846,11.8180816626378,12.8029218011909,
13.6836710227275),.UNSPECIFIED.);
#26981=B_SPLINE_CURVE_WITH_KNOTS('',3,(#455791,#455792,#455793,#455794,
#455795,#455796,#455797,#455798,#455799,#455800,#455801,#455802,#455803,
#455804,#455805,#455806,#455807,#455808,#455809,#455810,#455811,#455812,
#455813,#455814,#455815),.UNSPECIFIED.,.F.,.F.,(4,3,3,3,3,3,3,3,4),(-22.9424863416694,
-22.6513231867224,-21.6664830481693,-20.6816429096161,-19.696802771063,
-18.7119626325098,-17.7271224939567,-16.7422823554035,-16.6593010344898),
 .UNSPECIFIED.);
#26982=B_SPLINE_CURVE_WITH_KNOTS('',3,(#455816,#455817,#455818,#455819,
#455820,#455821,#455822,#455823,#455824,#455825,#455826,#455827,#455828,
#455829,#455830,#455831,#455832,#455833,#455834,#455835,#455836,#455837,
#455838,#455839,#455840),.UNSPECIFIED.,.F.,.F.,(4,3,3,3,3,3,3,3,4),(13.6836710227275,
13.7877619397441,14.7726020782972,15.7574422168504,16.7422823554035,17.7271224939567,
18.7119626325098,19.696802771063,19.966856329907),.UNSPECIFIED.);
#26983=B_SPLINE_CURVE_WITH_KNOTS('',3,(#455845,#455846,#455847,#455848,
#455849,#455850,#455851,#455852,#455853,#455854,#455855,#455856,#455857,
#455858,#455859,#455860,#455861,#455862,#455863,#455864,#455865,#455866),
 .UNSPECIFIED.,.F.,.F.,(4,3,3,3,3,3,3,4),(-29.225671648849,-28.5603640180413,
-27.5755238794882,-26.590683740935,-25.6058436023819,-24.6210034638287,
-23.6361633252756,-22.9424863416694),.UNSPECIFIED.);
#26984=B_SPLINE_CURVE_WITH_KNOTS('',3,(#455867,#455868,#455869,#455870,
#455871,#455872,#455873,#455874,#455875,#455876,#455877,#455878,#455879,
#455880,#455881,#455882,#455883,#455884,#455885,#455886,#455887,#455888),
 .UNSPECIFIED.,.F.,.F.,(4,3,3,3,3,3,3,4),(19.966856329907,20.6816429096161,
21.6664830481693,22.6513231867224,23.6361633252756,24.6210034638287,25.6058436023819,
26.2500416370866),.UNSPECIFIED.);
#26985=B_SPLINE_CURVE_WITH_KNOTS('',3,(#455894,#455895,#455896,#455897,
#455898,#455899),.UNSPECIFIED.,.F.,.F.,(4,1,1,4),(40.8407044966673,41.1602370044128,
42.1450771429659,43.0309593837163),.UNSPECIFIED.);
#26986=B_SPLINE_CURVE_WITH_KNOTS('',3,(#455902,#455903,#455904,#455905),
 .UNSPECIFIED.,.F.,.F.,(4,4),(40.8407044966673,41.7920422632082),
 .UNSPECIFIED.);
#26987=B_SPLINE_CURVE_WITH_KNOTS('',3,(#455910,#455911,#455912,#455913,
#455914,#455915,#455916,#455917,#455918,#455919),.UNSPECIFIED.,.F.,.F.,
(4,1,1,1,1,1,1,4),(34.5575191894877,35.2511961730939,36.236036311647,37.2208764502002,
38.2057165887533,39.1905567273065,40.1753968658596,40.8407044966673),
 .UNSPECIFIED.);
#26988=B_SPLINE_CURVE_WITH_KNOTS('',3,(#455920,#455921,#455922,#455923,
#455924,#455925,#455926,#455927,#455928,#455929,#455930),.UNSPECIFIED.,
 .F.,.F.,(4,1,1,1,1,1,1,1,4),(34.5575191894877,34.8981612933361,35.8830014318893,
36.8678415704424,37.8526817089956,38.8375218475487,39.8223619861019,40.807202124655,
40.8407044966673),.UNSPECIFIED.);
#26989=B_SPLINE_CURVE_WITH_KNOTS('',3,(#455935,#455936,#455937,#455938,
#455939,#455940,#455941,#455942,#455943,#455944,#455945),.UNSPECIFIED.,
 .F.,.F.,(4,1,1,1,1,1,1,1,4),(28.2743338823081,28.3573152032219,29.342155341775,
30.3269954803282,31.3118356188813,32.2966757574344,33.2815158959876,34.2663560345407,
34.5575191894877),.UNSPECIFIED.);
#26990=B_SPLINE_CURVE_WITH_KNOTS('',3,(#455946,#455947,#455948,#455949,
#455950,#455951,#455952,#455953,#455954,#455955),.UNSPECIFIED.,.F.,.F.,
(4,1,1,1,1,1,1,4),(28.2743338823081,28.9891204620172,29.9739606005704,30.9588007391235,
31.9436408776767,32.9284810162298,33.913321154783,34.5575191894877),
 .UNSPECIFIED.);
#26991=B_SPLINE_CURVE_WITH_KNOTS('',3,(#455960,#455961,#455962,#455963,
#455964,#455965,#455966,#455967,#455968,#455969),.UNSPECIFIED.,.F.,.F.,
(4,1,1,1,1,1,1,4),(21.9911485751285,22.448274371903,23.4331145104561,24.4179546490093,
25.4027947875624,26.3876349261156,27.3724750646687,28.2743338823081),
 .UNSPECIFIED.);
#26992=B_SPLINE_CURVE_WITH_KNOTS('',3,(#455970,#455971,#455972,#455973,
#455974,#455975,#455976,#455977,#455978,#455979,#455980),.UNSPECIFIED.,
 .F.,.F.,(4,1,1,1,1,1,1,1,4),(21.9911485751285,22.0952394921452,23.0800796306983,
24.0649197692515,25.0497599078046,26.0346000463578,27.0194401849109,28.0042803234641,
28.2743338823081),.UNSPECIFIED.);
#26993=B_SPLINE_CURVE_WITH_KNOTS('',3,(#455985,#455986,#455987,#455988,
#455989,#455990,#455991,#455992,#455993,#455994),.UNSPECIFIED.,.F.,.F.,
(4,1,1,1,1,1,1,4),(15.707963267949,16.5392335405841,17.5240736791372,18.5089138176904,
19.4937539562435,20.4785940947967,21.4634342333498,21.9911485751285),
 .UNSPECIFIED.);
#26994=B_SPLINE_CURVE_WITH_KNOTS('',3,(#455995,#455996,#455997,#455998,
#455999,#456000,#456001,#456002,#456003,#456004),.UNSPECIFIED.,.F.,.F.,
(4,1,1,1,1,1,1,4),(15.707963267949,16.1861986608263,17.1710387993794,18.1558789379326,
19.1407190764857,20.1255592150389,21.110399353592,21.9911485751285),
 .UNSPECIFIED.);
#26995=B_SPLINE_CURVE_WITH_KNOTS('',3,(#456154,#456155,#456156,#456157,
#456158,#456159,#456160,#456161,#456162,#456163,#456164,#456165,#456166,
#456167,#456168,#456169,#456170,#456171,#456172,#456173,#456174,#456175,
#456176,#456177,#456178,#456179,#456180,#456181,#456182,#456183,#456184,
#456185,#456186,#456187,#456188,#456189,#456190,#456191,#456192,#456193,
#456194,#456195,#456196,#456197,#456198,#456199,#456200,#456201,#456202,
#456203,#456204,#456205,#456206,#456207,#456208,#456209,#456210,#456211,
#456212,#456213,#456214,#456215,#456216,#456217,#456218,#456219,#456220,
#456221,#456222,#456223,#456224,#456225,#456226,#456227,#456228,#456229,
#456230,#456231,#456232,#456233,#456234,#456235,#456236,#456237,#456238,
#456239,#456240,#456241,#456242,#456243,#456244),.UNSPECIFIED.,.F.,.F.,
(4,3,3,3,3,3,3,3,3,3,3,3,3,3,3,3,3,3,3,3,3,3,3,3,3,3,3,3,3,3,4),(0.,0.0291704936873683,
0.0583901552072424,0.0892766589597223,0.102789504351432,0.112166362673238,
0.116534597984906,0.14527798460994,0.17392803078138,0.202083533954261,0.215008365363363,
0.220764604622565,0.22483118758101,0.252407730218333,0.279182155080764,
0.305482185227081,0.321094097925349,0.325435232071915,0.352007771215581,
0.37911010758988,0.405971172690074,0.418020595108885,0.425023905710974,
0.429595206514516,0.455898766278936,0.480742271809045,0.487658166045092,
0.494570770854422,0.519851794548597,0.544421019656577,0.55527278839937),
 .UNSPECIFIED.);
#26996=B_SPLINE_CURVE_WITH_KNOTS('',3,(#456245,#456246,#456247,#456248,
#456249,#456250,#456251,#456252,#456253,#456254,#456255,#456256,#456257,
#456258,#456259,#456260,#456261,#456262,#456263),.UNSPECIFIED.,.F.,.F.,
(4,3,3,3,3,3,4),(26.2500416370866,26.590683740935,27.5755238794882,28.5603640180413,
29.5452041565945,30.5300442951476,31.4159265358979),.UNSPECIFIED.);
#26997=B_SPLINE_CURVE_WITH_KNOTS('',3,(#456265,#456266,#456267,#456268,
#456269,#456270,#456271,#456272,#456273,#456274,#456275,#456276,#456277,
#456278,#456279,#456280,#456281,#456282,#456283,#456284,#456285,#456286,
#456287,#456288,#456289,#456290,#456291,#456292,#456293,#456294,#456295,
#456296,#456297,#456298,#456299,#456300,#456301,#456302,#456303,#456304,
#456305,#456306,#456307,#456308,#456309,#456310,#456311,#456312,#456313,
#456314,#456315,#456316,#456317,#456318,#456319,#456320,#456321,#456322,
#456323,#456324,#456325,#456326,#456327,#456328,#456329,#456330,#456331,
#456332,#456333,#456334,#456335,#456336,#456337,#456338,#456339,#456340,
#456341,#456342,#456343,#456344,#456345,#456346,#456347,#456348,#456349,
#456350,#456351,#456352,#456353,#456354,#456355),.UNSPECIFIED.,.F.,.F.,
(4,3,3,3,3,3,3,3,3,3,3,3,3,3,3,3,3,3,3,3,3,3,3,3,3,3,3,3,3,3,4),(0.,0.0238062091558073,
0.0483829200003844,0.0735693023851429,0.0861844508658027,0.0923222737131809,
0.09669810673984,0.122607870190124,0.149055649769671,0.175727680368522,
0.188356929884852,0.192627184956794,0.220007365861877,0.247709521968789,
0.2754116780757,0.285004370325409,0.293795122953647,0.298369842260591,0.325203400447931,
0.35364614768882,0.378533551524598,0.391516739337066,0.398116945812671,
0.403847639833503,0.432612326557626,0.462645589511981,0.47232137580103,
0.479347180528688,0.50891257055823,0.538120141855211,0.552745378375044),
 .UNSPECIFIED.);
#26998=B_SPLINE_CURVE_WITH_KNOTS('',3,(#456356,#456357,#456358,#456359,
#456360,#456361,#456362,#456363,#456364),.UNSPECIFIED.,.F.,.F.,(4,1,1,1,
1,1,4),(10.3761157273102,11.2619979680605,12.2468381066137,13.2316782451668,
14.21651838372,15.2013585222731,15.707963267949),.UNSPECIFIED.);
#26999=B_SPLINE_CURVE_WITH_KNOTS('',3,(#456368,#456369,#456370,#456371,
#456372,#456373,#456374,#456375),.UNSPECIFIED.,.F.,.F.,(4,1,1,1,1,4),(11.6150328478183,
12.5998729863715,13.5847131249246,14.5695532634778,15.5543934020309,15.707963267949),
 .UNSPECIFIED.);
#27000=B_SPLINE_CURVE_WITH_KNOTS('',3,(#456525,#456526,#456527,#456528,
#456529,#456530,#456531,#456532,#456533,#456534,#456535,#456536,#456537,
#456538,#456539,#456540,#456541,#456542,#456543,#456544,#456545,#456546,
#456547,#456548,#456549,#456550,#456551,#456552,#456553,#456554,#456555,
#456556,#456557,#456558,#456559,#456560,#456561,#456562,#456563,#456564,
#456565,#456566,#456567,#456568,#456569,#456570,#456571,#456572,#456573,
#456574,#456575,#456576,#456577,#456578,#456579,#456580,#456581,#456582,
#456583,#456584,#456585,#456586,#456587,#456588,#456589,#456590,#456591,
#456592,#456593,#456594,#456595,#456596,#456597,#456598,#456599,#456600,
#456601,#456602,#456603,#456604,#456605,#456606,#456607,#456608,#456609,
#456610,#456611,#456612,#456613,#456614,#456615),.UNSPECIFIED.,.F.,.F.,
(4,3,3,3,3,3,3,3,3,3,3,3,3,3,3,3,3,3,3,3,3,3,3,3,3,3,3,3,3,3,4),(0.,0.0238062091558071,
0.0483828706186186,0.0735692218797394,0.0861843753919871,0.0923221305421182,
0.0966981255468032,0.122607856296174,0.149055623017512,0.175727654618578,
0.18835688351681,0.192627137748861,0.220007313021443,0.247709495548573,
0.275411678075702,0.285004376041476,0.293795155716159,0.298369846935252,
0.325203393116049,0.353646141273424,0.378533545911127,0.391516729248669,
0.398116977240157,0.403847652647052,0.432612318543257,0.462645583501205,
0.472321362733173,0.479347182520809,0.508912572368484,0.538120187828272,
0.55274537837505),.UNSPECIFIED.);
#27001=B_SPLINE_CURVE_WITH_KNOTS('',3,(#456616,#456617,#456618,#456619,
#456620,#456621,#456622,#456623,#456624,#456625,#456626,#456627,#456628,
#456629,#456630,#456631,#456632,#456633,#456634,#456635,#456636,#456637,
#456638,#456639,#456640,#456641,#456642,#456643,#456644,#456645,#456646,
#456647,#456648,#456649,#456650,#456651,#456652,#456653,#456654,#456655,
#456656,#456657,#456658,#456659,#456660,#456661,#456662,#456663,#456664,
#456665,#456666,#456667,#456668,#456669,#456670,#456671,#456672,#456673,
#456674,#456675,#456676,#456677,#456678,#456679,#456680,#456681,#456682,
#456683,#456684,#456685,#456686,#456687,#456688,#456689,#456690,#456691,
#456692,#456693,#456694,#456695,#456696,#456697,#456698,#456699,#456700,
#456701,#456702,#456703,#456704,#456705,#456706),.UNSPECIFIED.,.F.,.F.,
(4,3,3,3,3,3,3,3,3,3,3,3,3,3,3,3,3,3,3,3,3,3,3,3,3,3,3,3,3,3,4),(0.,0.0291704936873701,
0.0583901514208582,0.0892766556466376,0.102789501245416,0.112166345743357,
0.116534589717914,0.145277976478382,0.173928009345204,0.20208347654446,
0.215008315129789,0.220764359590348,0.224831129685752,0.252407647279974,
0.279182017118223,0.305482185227093,0.321094097925361,0.325435232358679,
0.352007731597858,0.379110069176849,0.405971171510899,0.418020583618158,
0.42502391146057,0.42959521059718,0.455898797678682,0.480742295358858,0.487658257009521,
0.494570761890733,0.519851841940689,0.544421141195806,0.555272788399386),
 .UNSPECIFIED.);
#27002=B_SPLINE_CURVE_WITH_KNOTS('',3,(#456707,#456708,#456709,#456710,
#456711,#456712,#456713,#456714,#456715,#456716,#456717,#456718,#456719,
#456720,#456721,#456722),.UNSPECIFIED.,.F.,.F.,(4,3,3,3,3,4),(-33.4845647108071,
-32.4997245722539,-31.5148844337008,-30.5300442951476,-29.5452041565945,
-29.225671648849),.UNSPECIFIED.);
#27003=B_SPLINE_CURVE_WITH_KNOTS('',3,(#456732,#456733,#456734,#456735,
#456736,#456737,#456738,#456739,#456740,#456741,#456742,#456743,#456744,
#456745,#456746,#456747,#456748,#456749,#456750,#456751,#456752,#456753),
 .UNSPECIFIED.,.F.,.F.,(4,3,3,3,3,3,3,4),(-0.137266596901587,-0.120108272288889,
-0.114482300827285,-0.110524277642504,-0.080939047567984,-0.0517696842448276,
-0.0235157745135959,0.),.UNSPECIFIED.);
#27004=B_SPLINE_CURVE_WITH_KNOTS('',3,(#456755,#456756,#456757,#456758,
#456759,#456760,#456761,#456762,#456763,#456764,#456765,#456766,#456767,
#456768,#456769,#456770,#456771,#456772,#456773),.UNSPECIFIED.,.F.,.F.,
(4,3,3,3,3,3,4),(-0.658260979006767,-0.635315718400124,-0.606661307506358,
-0.584172758955614,-0.578302186585446,-0.54863415322041,-0.52069807482506),
 .UNSPECIFIED.);
#27005=B_SPLINE_CURVE_WITH_KNOTS('',3,(#457044,#457045,#457046,#457047,
#457048,#457049,#457050,#457051,#457052,#457053,#457054,#457055,#457056,
#457057,#457058,#457059,#457060,#457061,#457062,#457063,#457064,#457065,
#457066,#457067,#457068,#457069,#457070,#457071,#457072,#457073,#457074,
#457075,#457076,#457077,#457078,#457079,#457080,#457081,#457082,#457083,
#457084,#457085,#457086,#457087,#457088,#457089,#457090,#457091,#457092,
#457093,#457094,#457095,#457096,#457097,#457098,#457099,#457100,#457101,
#457102,#457103,#457104,#457105,#457106,#457107,#457108,#457109,#457110,
#457111,#457112,#457113),.UNSPECIFIED.,.F.,.F.,(4,3,3,3,3,3,3,3,3,3,3,3,
3,3,3,3,3,3,3,3,3,3,3,4),(0.,0.0272040286413901,0.0600270143818345,0.0934058988577766,
0.126267828410656,0.131862201401969,0.13651369641287,0.16911813316586,0.201670978277266,
0.233729929110374,0.249051354881678,0.259289013450942,0.263883210759706,
0.29536534390224,0.325978269163176,0.356301335280809,0.374706067837319,
0.381238410008019,0.386955324433938,0.417676149855772,0.448702433409449,
0.479505858091495,0.503539195732891,0.520698074825087),.UNSPECIFIED.);
#27006=B_SPLINE_CURVE_WITH_KNOTS('',3,(#457114,#457115,#457116,#457117,
#457118,#457119,#457120,#457121,#457122,#457123,#457124,#457125,#457126,
#457127,#457128,#457129),.UNSPECIFIED.,.F.,.F.,(4,3,3,3,3,4),(57.6650612733024,
57.6764209775632,58.6708420289005,59.6652630802378,60.6596841315751,61.57521601036),
 .UNSPECIFIED.);
#27007=B_SPLINE_CURVE_WITH_KNOTS('',3,(#457131,#457132,#457133,#457134,
#457135,#457136,#457137,#457138,#457139,#457140,#457141,#457142,#457143,
#457144,#457145,#457146,#457147,#457148,#457149,#457150,#457151,#457152,
#457153,#457154,#457155,#457156,#457157,#457158,#457159,#457160,#457161,
#457162,#457163,#457164,#457165,#457166,#457167,#457168,#457169,#457170,
#457171,#457172,#457173,#457174,#457175,#457176,#457177,#457178,#457179,
#457180,#457181,#457182,#457183,#457184,#457185,#457186,#457187,#457188,
#457189,#457190,#457191,#457192,#457193,#457194,#457195,#457196,#457197,
#457198,#457199,#457200,#457201,#457202,#457203,#457204,#457205,#457206,
#457207,#457208,#457209,#457210,#457211,#457212,#457213,#457214,#457215,
#457216,#457217,#457218),.UNSPECIFIED.,.F.,.F.,(4,3,3,3,3,3,3,3,3,3,3,3,
3,3,3,3,3,3,3,3,3,3,3,3,3,3,3,3,3,4),(0.,0.0228820365931952,0.051218373414923,
0.080268233877054,0.111010300783671,0.116758747556016,0.146658127377976,
0.177121111126461,0.207780701795497,0.222583710212308,0.229317438129826,
0.234676157420321,0.26606503457775,0.297281607920556,0.326204769129986,
0.346801497054257,0.352594205912184,0.356892740676827,0.387479019349114,
0.41883328811469,0.450858933696391,0.476470618974131,0.482836412282282,
0.515509333257769,0.548396254053967,0.563515013889454,0.570640443970302,
0.604038137402537,0.636956540638902,0.655752415918318),.UNSPECIFIED.);
#27008=B_SPLINE_CURVE_WITH_KNOTS('',3,(#457219,#457220,#457221,#457222,
#457223,#457224,#457225,#457226,#457227),.UNSPECIFIED.,.F.,.F.,(4,1,1,1,
1,1,4),(10.3761157273102,11.2916476060951,12.2860686574324,13.2804897087697,
14.2749107601069,15.2693318114442,15.7079632679489),.UNSPECIFIED.);
#27009=B_SPLINE_CURVE_WITH_KNOTS('',3,(#457231,#457232,#457233,#457234,
#457235,#457236,#457237,#457238),.UNSPECIFIED.,.F.,.F.,(4,1,1,1,1,4),(11.6150328478183,
12.6094538991556,13.6038749504929,14.5982960018302,15.5927170531675,15.7079632679489),
 .UNSPECIFIED.);
#27010=B_SPLINE_CURVE_WITH_KNOTS('',3,(#457507,#457508,#457509,#457510,
#457511,#457512,#457513,#457514,#457515,#457516,#457517,#457518,#457519,
#457520,#457521,#457522,#457523,#457524,#457525,#457526,#457527,#457528,
#457529,#457530,#457531,#457532,#457533,#457534,#457535,#457536,#457537,
#457538,#457539,#457540,#457541,#457542,#457543,#457544,#457545,#457546,
#457547,#457548,#457549,#457550,#457551,#457552,#457553,#457554,#457555,
#457556,#457557,#457558,#457559,#457560,#457561,#457562,#457563,#457564,
#457565,#457566,#457567,#457568,#457569,#457570,#457571,#457572,#457573,
#457574,#457575,#457576,#457577,#457578,#457579,#457580,#457581,#457582,
#457583,#457584,#457585,#457586,#457587,#457588,#457589,#457590,#457591,
#457592,#457593,#457594,#457595,#457596,#457597,#457598,#457599,#457600),
 .UNSPECIFIED.,.F.,.F.,(4,3,3,3,3,3,3,3,3,3,3,3,3,3,3,3,3,3,3,3,3,3,3,3,
3,3,3,3,3,3,3,4),(0.,0.0272040286413987,0.0600270092260691,0.0934058933249245,
0.126267823569411,0.131862171516485,0.13651368729204,0.169118124243381,
0.201670964051155,0.233729898345333,0.249051327962268,0.259288987827642,
0.263883168763017,0.295365290437433,0.325978188171709,0.356301335280814,
0.375173813013688,0.383411475909621,0.388182941704446,0.418653739168425,
0.449704751396772,0.480514094750049,0.494157308726131,0.502507051908377,
0.507342387999586,0.537640987329864,0.567795985249096,0.576607688145916,
0.582412660202483,0.611714236442306,0.640195300747252,0.658260979006793),
 .UNSPECIFIED.);
#27011=B_SPLINE_CURVE_WITH_KNOTS('',3,(#457602,#457603,#457604,#457605,
#457606,#457607,#457608,#457609,#457610,#457611,#457612,#457613,#457614),
 .UNSPECIFIED.,.F.,.F.,(4,3,3,3,4),(-63.642947285587,-62.6485262342497,
-61.6541051829124,-60.6596841315751,-60.641598184747),.UNSPECIFIED.);
#27012=B_SPLINE_CURVE_WITH_KNOTS('',3,(#457615,#457616,#457617,#457618,
#457619,#457620,#457621,#457622,#457623,#457624,#457625,#457626,#457627,
#457628,#457629,#457630,#457631,#457632,#457633,#457634,#457635,#457636,
#457637,#457638,#457639,#457640,#457641,#457642,#457643,#457644,#457645,
#457646,#457647,#457648,#457649,#457650,#457651,#457652,#457653,#457654,
#457655,#457656,#457657,#457658,#457659,#457660,#457661,#457662,#457663,
#457664,#457665,#457666,#457667,#457668,#457669,#457670,#457671,#457672,
#457673,#457674,#457675,#457676,#457677,#457678,#457679,#457680,#457681),
 .UNSPECIFIED.,.F.,.F.,(4,3,3,3,3,3,3,3,3,3,3,3,3,3,3,3,3,3,3,3,3,3,4),
(0.137266596905892,0.167584419985923,0.198231972141458,0.230225171388588,
0.234597263271361,0.265985606555594,0.297202865015363,0.326204769129979,
0.346801497054249,0.352594207537935,0.356892744389492,0.387479014259225,
0.418833269879323,0.450858809182976,0.476470510024891,0.482836382836457,
0.51550929223882,0.548396212827012,0.563514950346987,0.570640427639483,
0.604038123799383,0.636956554307592,0.6557524159183),.UNSPECIFIED.);
#30704=LINE('',#454969,#34506);
#30705=LINE('',#454993,#34507);
#30706=LINE('',#455041,#34508);
#30707=LINE('',#455089,#34509);
#30708=LINE('',#455143,#34510);
#30709=LINE('',#455191,#34511);
#30710=LINE('',#455239,#34512);
#30711=LINE('',#455293,#34513);
#30712=LINE('',#455341,#34514);
#30713=LINE('',#455389,#34515);
#30714=LINE('',#455437,#34516);
#30715=LINE('',#455448,#34517);
#30716=LINE('',#455474,#34518);
#30717=LINE('',#455498,#34519);
#30718=LINE('',#455522,#34520);
#30719=LINE('',#455547,#34521);
#30720=LINE('',#455572,#34522);
#30721=LINE('',#455596,#34523);
#30722=LINE('',#455621,#34524);
#30723=LINE('',#455646,#34525);
#30724=LINE('',#455670,#34526);
#30725=LINE('',#455694,#34527);
#30726=LINE('',#455742,#34528);
#30727=LINE('',#455790,#34529);
#30728=LINE('',#455844,#34530);
#30729=LINE('',#455892,#34531);
#30730=LINE('',#455909,#34532);
#30731=LINE('',#455934,#34533);
#30732=LINE('',#455959,#34534);
#30733=LINE('',#455984,#34535);
#30734=LINE('',#457688,#34536);
#30735=LINE('',#457693,#34537);
#30736=LINE('',#457697,#34538);
#30737=LINE('',#457703,#34539);
#30738=LINE('',#457708,#34540);
#30739=LINE('',#457712,#34541);
#34506=VECTOR('',#130154,3.5);
#34507=VECTOR('',#130159,3.5);
#34508=VECTOR('',#130162,3.5);
#34509=VECTOR('',#130165,3.5);
#34510=VECTOR('',#130168,3.5);
#34511=VECTOR('',#130171,3.5);
#34512=VECTOR('',#130174,3.5);
#34513=VECTOR('',#130177,3.5);
#34514=VECTOR('',#130180,3.5);
#34515=VECTOR('',#130183,3.5);
#34516=VECTOR('',#130186,2.872);
#34517=VECTOR('',#130191,2.872);
#34518=VECTOR('',#130196,2.872);
#34519=VECTOR('',#130199,2.872);
#34520=VECTOR('',#130202,2.872);
#34521=VECTOR('',#130205,2.872);
#34522=VECTOR('',#130208,2.872);
#34523=VECTOR('',#130211,2.872);
#34524=VECTOR('',#130214,2.872);
#34525=VECTOR('',#130217,2.872);
#34526=VECTOR('',#130220,3.);
#34527=VECTOR('',#130225,3.);
#34528=VECTOR('',#130228,3.);
#34529=VECTOR('',#130231,3.);
#34530=VECTOR('',#130234,3.);
#34531=VECTOR('',#130237,2.37175);
#34532=VECTOR('',#130242,2.37175);
#34533=VECTOR('',#130245,2.37175);
#34534=VECTOR('',#130248,2.37175);
#34535=VECTOR('',#130251,2.37175);
#34536=VECTOR('',#130280,2.5);
#34537=VECTOR('',#130287,1.4);
#34538=VECTOR('',#130294,3.);
#34539=VECTOR('',#130301,2.1);
#34540=VECTOR('',#130308,2.1);
#34541=VECTOR('',#130313,1.);
#43319=VERTEX_POINT('',#454967);
#43320=VERTEX_POINT('',#454968);
#43321=VERTEX_POINT('',#454970);
#43322=VERTEX_POINT('',#454981);
#43323=VERTEX_POINT('',#454991);
#43324=VERTEX_POINT('',#454992);
#43325=VERTEX_POINT('',#455039);
#43326=VERTEX_POINT('',#455040);
#43327=VERTEX_POINT('',#455087);
#43328=VERTEX_POINT('',#455088);
#43329=VERTEX_POINT('',#455141);
#43330=VERTEX_POINT('',#455142);
#43331=VERTEX_POINT('',#455189);
#43332=VERTEX_POINT('',#455190);
#43333=VERTEX_POINT('',#455237);
#43334=VERTEX_POINT('',#455238);
#43335=VERTEX_POINT('',#455291);
#43336=VERTEX_POINT('',#455292);
#43337=VERTEX_POINT('',#455339);
#43338=VERTEX_POINT('',#455340);
#43339=VERTEX_POINT('',#455387);
#43340=VERTEX_POINT('',#455388);
#43341=VERTEX_POINT('',#455435);
#43342=VERTEX_POINT('',#455436);
#43343=VERTEX_POINT('',#455438);
#43344=VERTEX_POINT('',#455446);
#43345=VERTEX_POINT('',#455447);
#43346=VERTEX_POINT('',#455459);
#43347=VERTEX_POINT('',#455472);
#43348=VERTEX_POINT('',#455473);
#43349=VERTEX_POINT('',#455496);
#43350=VERTEX_POINT('',#455497);
#43351=VERTEX_POINT('',#455520);
#43352=VERTEX_POINT('',#455521);
#43353=VERTEX_POINT('',#455545);
#43354=VERTEX_POINT('',#455546);
#43355=VERTEX_POINT('',#455570);
#43356=VERTEX_POINT('',#455571);
#43357=VERTEX_POINT('',#455594);
#43358=VERTEX_POINT('',#455595);
#43359=VERTEX_POINT('',#455619);
#43360=VERTEX_POINT('',#455620);
#43361=VERTEX_POINT('',#455644);
#43362=VERTEX_POINT('',#455645);
#43363=VERTEX_POINT('',#455668);
#43364=VERTEX_POINT('',#455669);
#43365=VERTEX_POINT('',#455671);
#43366=VERTEX_POINT('',#455682);
#43367=VERTEX_POINT('',#455692);
#43368=VERTEX_POINT('',#455693);
#43369=VERTEX_POINT('',#455740);
#43370=VERTEX_POINT('',#455741);
#43371=VERTEX_POINT('',#455788);
#43372=VERTEX_POINT('',#455789);
#43373=VERTEX_POINT('',#455842);
#43374=VERTEX_POINT('',#455843);
#43375=VERTEX_POINT('',#455890);
#43376=VERTEX_POINT('',#455891);
#43377=VERTEX_POINT('',#455893);
#43378=VERTEX_POINT('',#455900);
#43379=VERTEX_POINT('',#455907);
#43380=VERTEX_POINT('',#455908);
#43381=VERTEX_POINT('',#455932);
#43382=VERTEX_POINT('',#455933);
#43383=VERTEX_POINT('',#455957);
#43384=VERTEX_POINT('',#455958);
#43385=VERTEX_POINT('',#455982);
#43386=VERTEX_POINT('',#455983);
#43387=VERTEX_POINT('',#456153);
#43388=VERTEX_POINT('',#456264);
#43389=VERTEX_POINT('',#456366);
#43390=VERTEX_POINT('',#456524);
#43391=VERTEX_POINT('',#456725);
#43392=VERTEX_POINT('',#456729);
#43393=VERTEX_POINT('',#456730);
#43394=VERTEX_POINT('',#456754);
#43395=VERTEX_POINT('',#457043);
#43396=VERTEX_POINT('',#457130);
#43397=VERTEX_POINT('',#457229);
#43398=VERTEX_POINT('',#457601);
#43399=VERTEX_POINT('',#457683);
#43400=VERTEX_POINT('',#457684);
#43401=VERTEX_POINT('',#457687);
#43402=VERTEX_POINT('',#457691);
#43403=VERTEX_POINT('',#457700);
#43404=VERTEX_POINT('',#457702);
#43405=VERTEX_POINT('',#457706);
#43406=VERTEX_POINT('',#457710);
#57716=EDGE_CURVE('',#43319,#43320,#30704,.T.);
#57717=EDGE_CURVE('',#43319,#43321,#26936,.T.);
#57718=EDGE_CURVE('',#43321,#43322,#23442,.F.);
#57719=EDGE_CURVE('',#43322,#43320,#26937,.T.);
#57720=EDGE_CURVE('',#43323,#43324,#30705,.T.);
#57721=EDGE_CURVE('',#43323,#43319,#26938,.T.);
#57722=EDGE_CURVE('',#43320,#43324,#26939,.T.);
#57723=EDGE_CURVE('',#43325,#43326,#30706,.T.);
#57724=EDGE_CURVE('',#43325,#43323,#26940,.T.);
#57725=EDGE_CURVE('',#43324,#43326,#26941,.T.);
#57726=EDGE_CURVE('',#43327,#43328,#30707,.T.);
#57727=EDGE_CURVE('',#43327,#43325,#26942,.T.);
#57728=EDGE_CURVE('',#43326,#43328,#26943,.T.);
#57729=EDGE_CURVE('',#43329,#43330,#30708,.T.);
#57730=EDGE_CURVE('',#43329,#43327,#26944,.T.);
#57731=EDGE_CURVE('',#43328,#43330,#26945,.T.);
#57732=EDGE_CURVE('',#43331,#43332,#30709,.T.);
#57733=EDGE_CURVE('',#43331,#43329,#26946,.T.);
#57734=EDGE_CURVE('',#43330,#43332,#26947,.T.);
#57735=EDGE_CURVE('',#43333,#43334,#30710,.T.);
#57736=EDGE_CURVE('',#43333,#43331,#26948,.T.);
#57737=EDGE_CURVE('',#43332,#43334,#26949,.T.);
#57738=EDGE_CURVE('',#43335,#43336,#30711,.T.);
#57739=EDGE_CURVE('',#43335,#43333,#26950,.T.);
#57740=EDGE_CURVE('',#43334,#43336,#26951,.T.);
#57741=EDGE_CURVE('',#43337,#43338,#30712,.T.);
#57742=EDGE_CURVE('',#43337,#43335,#26952,.T.);
#57743=EDGE_CURVE('',#43336,#43338,#26953,.T.);
#57744=EDGE_CURVE('',#43339,#43340,#30713,.T.);
#57745=EDGE_CURVE('',#43339,#43337,#26954,.T.);
#57746=EDGE_CURVE('',#43338,#43340,#26955,.T.);
#57747=EDGE_CURVE('',#43341,#43342,#30714,.T.);
#57748=EDGE_CURVE('',#43341,#43343,#26956,.T.);
#57749=EDGE_CURVE('',#43342,#43343,#23443,.T.);
#57750=EDGE_CURVE('',#43344,#43345,#30715,.T.);
#57751=EDGE_CURVE('',#43344,#43341,#26957,.T.);
#57752=EDGE_CURVE('',#43346,#43342,#23444,.T.);
#57753=EDGE_CURVE('',#43345,#43346,#26958,.T.);
#57754=EDGE_CURVE('',#43347,#43348,#30716,.T.);
#57755=EDGE_CURVE('',#43347,#43344,#26959,.T.);
#57756=EDGE_CURVE('',#43348,#43345,#26960,.T.);
#57757=EDGE_CURVE('',#43349,#43350,#30717,.T.);
#57758=EDGE_CURVE('',#43349,#43347,#26961,.T.);
#57759=EDGE_CURVE('',#43350,#43348,#26962,.T.);
#57760=EDGE_CURVE('',#43351,#43352,#30718,.T.);
#57761=EDGE_CURVE('',#43351,#43349,#26963,.T.);
#57762=EDGE_CURVE('',#43352,#43350,#26964,.T.);
#57763=EDGE_CURVE('',#43353,#43354,#30719,.T.);
#57764=EDGE_CURVE('',#43353,#43351,#26965,.T.);
#57765=EDGE_CURVE('',#43354,#43352,#26966,.T.);
#57766=EDGE_CURVE('',#43355,#43356,#30720,.T.);
#57767=EDGE_CURVE('',#43355,#43353,#26967,.T.);
#57768=EDGE_CURVE('',#43356,#43354,#26968,.T.);
#57769=EDGE_CURVE('',#43357,#43358,#30721,.T.);
#57770=EDGE_CURVE('',#43357,#43355,#26969,.T.);
#57771=EDGE_CURVE('',#43358,#43356,#26970,.T.);
#57772=EDGE_CURVE('',#43359,#43360,#30722,.T.);
#57773=EDGE_CURVE('',#43359,#43357,#26971,.T.);
#57774=EDGE_CURVE('',#43360,#43358,#26972,.T.);
#57775=EDGE_CURVE('',#43361,#43362,#30723,.T.);
#57776=EDGE_CURVE('',#43361,#43359,#26973,.T.);
#57777=EDGE_CURVE('',#43362,#43360,#26974,.T.);
#57778=EDGE_CURVE('',#43363,#43364,#30724,.T.);
#57779=EDGE_CURVE('',#43363,#43365,#26975,.T.);
#57780=EDGE_CURVE('',#43366,#43365,#23445,.T.);
#57781=EDGE_CURVE('',#43366,#43364,#26976,.T.);
#57782=EDGE_CURVE('',#43367,#43368,#30725,.T.);
#57783=EDGE_CURVE('',#43367,#43363,#26977,.T.);
#57784=EDGE_CURVE('',#43364,#43368,#26978,.T.);
#57785=EDGE_CURVE('',#43369,#43370,#30726,.T.);
#57786=EDGE_CURVE('',#43369,#43367,#26979,.T.);
#57787=EDGE_CURVE('',#43368,#43370,#26980,.T.);
#57788=EDGE_CURVE('',#43371,#43372,#30727,.T.);
#57789=EDGE_CURVE('',#43371,#43369,#26981,.T.);
#57790=EDGE_CURVE('',#43370,#43372,#26982,.T.);
#57791=EDGE_CURVE('',#43373,#43374,#30728,.T.);
#57792=EDGE_CURVE('',#43373,#43371,#26983,.T.);
#57793=EDGE_CURVE('',#43372,#43374,#26984,.T.);
#57794=EDGE_CURVE('',#43375,#43376,#30729,.T.);
#57795=EDGE_CURVE('',#43375,#43377,#26985,.T.);
#57796=EDGE_CURVE('',#43378,#43377,#23446,.T.);
#57797=EDGE_CURVE('',#43376,#43378,#26986,.T.);
#57798=EDGE_CURVE('',#43379,#43380,#30730,.T.);
#57799=EDGE_CURVE('',#43379,#43375,#26987,.T.);
#57800=EDGE_CURVE('',#43380,#43376,#26988,.T.);
#57801=EDGE_CURVE('',#43381,#43382,#30731,.T.);
#57802=EDGE_CURVE('',#43381,#43379,#26989,.T.);
#57803=EDGE_CURVE('',#43382,#43380,#26990,.T.);
#57804=EDGE_CURVE('',#43383,#43384,#30732,.T.);
#57805=EDGE_CURVE('',#43383,#43381,#26991,.T.);
#57806=EDGE_CURVE('',#43384,#43382,#26992,.T.);
#57807=EDGE_CURVE('',#43385,#43386,#30733,.T.);
#57808=EDGE_CURVE('',#43385,#43383,#26993,.T.);
#57809=EDGE_CURVE('',#43386,#43384,#26994,.T.);
#57810=EDGE_CURVE('',#43387,#43378,#26995,.T.);
#57811=EDGE_CURVE('',#43374,#43387,#26996,.T.);
#57812=EDGE_CURVE('',#43388,#43366,#26997,.T.);
#57813=EDGE_CURVE('',#43388,#43386,#26998,.T.);
#57814=EDGE_CURVE('',#43389,#43388,#23447,.T.);
#57815=EDGE_CURVE('',#43389,#43385,#26999,.T.);
#57816=EDGE_CURVE('',#43377,#43390,#27000,.T.);
#57817=EDGE_CURVE('',#43365,#43389,#27001,.T.);
#57818=EDGE_CURVE('',#43390,#43373,#27002,.T.);
#57819=EDGE_CURVE('',#43390,#43387,#23448,.T.);
#57820=EDGE_CURVE('',#43391,#43391,#23449,.T.);
#57821=EDGE_CURVE('',#43392,#43393,#23450,.T.);
#57822=EDGE_CURVE('',#43392,#43346,#27003,.T.);
#57823=EDGE_CURVE('',#43343,#43394,#27004,.T.);
#57824=EDGE_CURVE('',#43393,#43394,#23451,.T.);
#57825=EDGE_CURVE('',#43395,#43392,#27005,.T.);
#57826=EDGE_CURVE('',#43340,#43395,#27006,.T.);
#57827=EDGE_CURVE('',#43396,#43322,#27007,.T.);
#57828=EDGE_CURVE('',#43396,#43362,#27008,.T.);
#57829=EDGE_CURVE('',#43397,#43396,#23452,.T.);
#57830=EDGE_CURVE('',#43397,#43361,#27009,.T.);
#57831=EDGE_CURVE('',#43321,#43397,#27010,.T.);
#57832=EDGE_CURVE('',#43398,#43339,#27011,.T.);
#57833=EDGE_CURVE('',#43394,#43398,#27012,.T.);
#57834=EDGE_CURVE('',#43399,#43400,#23453,.T.);
#57835=EDGE_CURVE('',#43400,#43399,#23454,.T.);
#57836=EDGE_CURVE('',#43400,#43401,#30734,.T.);
#57837=EDGE_CURVE('',#43401,#43401,#23455,.T.);
#57838=EDGE_CURVE('',#43402,#43402,#23456,.T.);
#57839=EDGE_CURVE('',#43402,#43391,#30735,.T.);
#57840=EDGE_CURVE('',#43398,#43395,#23457,.T.);
#57841=EDGE_CURVE('',#43399,#43393,#30736,.T.);
#57842=EDGE_CURVE('',#43394,#43392,#23458,.T.);
#57843=EDGE_CURVE('',#43403,#43403,#23459,.T.);
#57844=EDGE_CURVE('',#43403,#43404,#30737,.T.);
#57845=EDGE_CURVE('',#43404,#43404,#23460,.T.);
#57846=EDGE_CURVE('',#43405,#43405,#23461,.T.);
#57847=EDGE_CURVE('',#43405,#43403,#30738,.T.);
#57848=EDGE_CURVE('',#43406,#43406,#23462,.T.);
#57849=EDGE_CURVE('',#43406,#43405,#30739,.T.);
#86428=ORIENTED_EDGE('',*,*,#57716,.F.);
#86429=ORIENTED_EDGE('',*,*,#57717,.T.);
#86430=ORIENTED_EDGE('',*,*,#57718,.T.);
#86431=ORIENTED_EDGE('',*,*,#57719,.T.);
#86432=ORIENTED_EDGE('',*,*,#57720,.F.);
#86433=ORIENTED_EDGE('',*,*,#57721,.T.);
#86434=ORIENTED_EDGE('',*,*,#57716,.T.);
#86435=ORIENTED_EDGE('',*,*,#57722,.T.);
#86436=ORIENTED_EDGE('',*,*,#57723,.F.);
#86437=ORIENTED_EDGE('',*,*,#57724,.T.);
#86438=ORIENTED_EDGE('',*,*,#57720,.T.);
#86439=ORIENTED_EDGE('',*,*,#57725,.T.);
#86440=ORIENTED_EDGE('',*,*,#57726,.F.);
#86441=ORIENTED_EDGE('',*,*,#57727,.T.);
#86442=ORIENTED_EDGE('',*,*,#57723,.T.);
#86443=ORIENTED_EDGE('',*,*,#57728,.T.);
#86444=ORIENTED_EDGE('',*,*,#57729,.F.);
#86445=ORIENTED_EDGE('',*,*,#57730,.T.);
#86446=ORIENTED_EDGE('',*,*,#57726,.T.);
#86447=ORIENTED_EDGE('',*,*,#57731,.T.);
#86448=ORIENTED_EDGE('',*,*,#57732,.F.);
#86449=ORIENTED_EDGE('',*,*,#57733,.T.);
#86450=ORIENTED_EDGE('',*,*,#57729,.T.);
#86451=ORIENTED_EDGE('',*,*,#57734,.T.);
#86452=ORIENTED_EDGE('',*,*,#57735,.F.);
#86453=ORIENTED_EDGE('',*,*,#57736,.T.);
#86454=ORIENTED_EDGE('',*,*,#57732,.T.);
#86455=ORIENTED_EDGE('',*,*,#57737,.T.);
#86456=ORIENTED_EDGE('',*,*,#57738,.F.);
#86457=ORIENTED_EDGE('',*,*,#57739,.T.);
#86458=ORIENTED_EDGE('',*,*,#57735,.T.);
#86459=ORIENTED_EDGE('',*,*,#57740,.T.);
#86460=ORIENTED_EDGE('',*,*,#57741,.F.);
#86461=ORIENTED_EDGE('',*,*,#57742,.T.);
#86462=ORIENTED_EDGE('',*,*,#57738,.T.);
#86463=ORIENTED_EDGE('',*,*,#57743,.T.);
#86464=ORIENTED_EDGE('',*,*,#57744,.F.);
#86465=ORIENTED_EDGE('',*,*,#57745,.T.);
#86466=ORIENTED_EDGE('',*,*,#57741,.T.);
#86467=ORIENTED_EDGE('',*,*,#57746,.T.);
#86468=ORIENTED_EDGE('',*,*,#57747,.F.);
#86469=ORIENTED_EDGE('',*,*,#57748,.T.);
#86470=ORIENTED_EDGE('',*,*,#57749,.F.);
#86471=ORIENTED_EDGE('',*,*,#57750,.F.);
#86472=ORIENTED_EDGE('',*,*,#57751,.T.);
#86473=ORIENTED_EDGE('',*,*,#57747,.T.);
#86474=ORIENTED_EDGE('',*,*,#57752,.F.);
#86475=ORIENTED_EDGE('',*,*,#57753,.F.);
#86476=ORIENTED_EDGE('',*,*,#57754,.F.);
#86477=ORIENTED_EDGE('',*,*,#57755,.T.);
#86478=ORIENTED_EDGE('',*,*,#57750,.T.);
#86479=ORIENTED_EDGE('',*,*,#57756,.F.);
#86480=ORIENTED_EDGE('',*,*,#57757,.F.);
#86481=ORIENTED_EDGE('',*,*,#57758,.T.);
#86482=ORIENTED_EDGE('',*,*,#57754,.T.);
#86483=ORIENTED_EDGE('',*,*,#57759,.F.);
#86484=ORIENTED_EDGE('',*,*,#57760,.F.);
#86485=ORIENTED_EDGE('',*,*,#57761,.T.);
#86486=ORIENTED_EDGE('',*,*,#57757,.T.);
#86487=ORIENTED_EDGE('',*,*,#57762,.F.);
#86488=ORIENTED_EDGE('',*,*,#57763,.F.);
#86489=ORIENTED_EDGE('',*,*,#57764,.T.);
#86490=ORIENTED_EDGE('',*,*,#57760,.T.);
#86491=ORIENTED_EDGE('',*,*,#57765,.F.);
#86492=ORIENTED_EDGE('',*,*,#57766,.F.);
#86493=ORIENTED_EDGE('',*,*,#57767,.T.);
#86494=ORIENTED_EDGE('',*,*,#57763,.T.);
#86495=ORIENTED_EDGE('',*,*,#57768,.F.);
#86496=ORIENTED_EDGE('',*,*,#57769,.F.);
#86497=ORIENTED_EDGE('',*,*,#57770,.T.);
#86498=ORIENTED_EDGE('',*,*,#57766,.T.);
#86499=ORIENTED_EDGE('',*,*,#57771,.F.);
#86500=ORIENTED_EDGE('',*,*,#57772,.F.);
#86501=ORIENTED_EDGE('',*,*,#57773,.T.);
#86502=ORIENTED_EDGE('',*,*,#57769,.T.);
#86503=ORIENTED_EDGE('',*,*,#57774,.F.);
#86504=ORIENTED_EDGE('',*,*,#57775,.F.);
#86505=ORIENTED_EDGE('',*,*,#57776,.T.);
#86506=ORIENTED_EDGE('',*,*,#57772,.T.);
#86507=ORIENTED_EDGE('',*,*,#57777,.F.);
#86508=ORIENTED_EDGE('',*,*,#57778,.F.);
#86509=ORIENTED_EDGE('',*,*,#57779,.T.);
#86510=ORIENTED_EDGE('',*,*,#57780,.F.);
#86511=ORIENTED_EDGE('',*,*,#57781,.T.);
#86512=ORIENTED_EDGE('',*,*,#57782,.F.);
#86513=ORIENTED_EDGE('',*,*,#57783,.T.);
#86514=ORIENTED_EDGE('',*,*,#57778,.T.);
#86515=ORIENTED_EDGE('',*,*,#57784,.T.);
#86516=ORIENTED_EDGE('',*,*,#57785,.F.);
#86517=ORIENTED_EDGE('',*,*,#57786,.T.);
#86518=ORIENTED_EDGE('',*,*,#57782,.T.);
#86519=ORIENTED_EDGE('',*,*,#57787,.T.);
#86520=ORIENTED_EDGE('',*,*,#57788,.F.);
#86521=ORIENTED_EDGE('',*,*,#57789,.T.);
#86522=ORIENTED_EDGE('',*,*,#57785,.T.);
#86523=ORIENTED_EDGE('',*,*,#57790,.T.);
#86524=ORIENTED_EDGE('',*,*,#57791,.F.);
#86525=ORIENTED_EDGE('',*,*,#57792,.T.);
#86526=ORIENTED_EDGE('',*,*,#57788,.T.);
#86527=ORIENTED_EDGE('',*,*,#57793,.T.);
#86528=ORIENTED_EDGE('',*,*,#57794,.F.);
#86529=ORIENTED_EDGE('',*,*,#57795,.T.);
#86530=ORIENTED_EDGE('',*,*,#57796,.F.);
#86531=ORIENTED_EDGE('',*,*,#57797,.F.);
#86532=ORIENTED_EDGE('',*,*,#57798,.F.);
#86533=ORIENTED_EDGE('',*,*,#57799,.T.);
#86534=ORIENTED_EDGE('',*,*,#57794,.T.);
#86535=ORIENTED_EDGE('',*,*,#57800,.F.);
#86536=ORIENTED_EDGE('',*,*,#57801,.F.);
#86537=ORIENTED_EDGE('',*,*,#57802,.T.);
#86538=ORIENTED_EDGE('',*,*,#57798,.T.);
#86539=ORIENTED_EDGE('',*,*,#57803,.F.);
#86540=ORIENTED_EDGE('',*,*,#57804,.F.);
#86541=ORIENTED_EDGE('',*,*,#57805,.T.);
#86542=ORIENTED_EDGE('',*,*,#57801,.T.);
#86543=ORIENTED_EDGE('',*,*,#57806,.F.);
#86544=ORIENTED_EDGE('',*,*,#57807,.F.);
#86545=ORIENTED_EDGE('',*,*,#57808,.T.);
#86546=ORIENTED_EDGE('',*,*,#57804,.T.);
#86547=ORIENTED_EDGE('',*,*,#57809,.F.);
#86548=ORIENTED_EDGE('',*,*,#57810,.F.);
#86549=ORIENTED_EDGE('',*,*,#57811,.F.);
#86550=ORIENTED_EDGE('',*,*,#57793,.F.);
#86551=ORIENTED_EDGE('',*,*,#57790,.F.);
#86552=ORIENTED_EDGE('',*,*,#57787,.F.);
#86553=ORIENTED_EDGE('',*,*,#57784,.F.);
#86554=ORIENTED_EDGE('',*,*,#57781,.F.);
#86555=ORIENTED_EDGE('',*,*,#57812,.F.);
#86556=ORIENTED_EDGE('',*,*,#57813,.T.);
#86557=ORIENTED_EDGE('',*,*,#57809,.T.);
#86558=ORIENTED_EDGE('',*,*,#57806,.T.);
#86559=ORIENTED_EDGE('',*,*,#57803,.T.);
#86560=ORIENTED_EDGE('',*,*,#57800,.T.);
#86561=ORIENTED_EDGE('',*,*,#57797,.T.);
#86562=ORIENTED_EDGE('',*,*,#57807,.T.);
#86563=ORIENTED_EDGE('',*,*,#57813,.F.);
#86564=ORIENTED_EDGE('',*,*,#57814,.F.);
#86565=ORIENTED_EDGE('',*,*,#57815,.T.);
#86566=ORIENTED_EDGE('',*,*,#57816,.F.);
#86567=ORIENTED_EDGE('',*,*,#57795,.F.);
#86568=ORIENTED_EDGE('',*,*,#57799,.F.);
#86569=ORIENTED_EDGE('',*,*,#57802,.F.);
#86570=ORIENTED_EDGE('',*,*,#57805,.F.);
#86571=ORIENTED_EDGE('',*,*,#57808,.F.);
#86572=ORIENTED_EDGE('',*,*,#57815,.F.);
#86573=ORIENTED_EDGE('',*,*,#57817,.F.);
#86574=ORIENTED_EDGE('',*,*,#57779,.F.);
#86575=ORIENTED_EDGE('',*,*,#57783,.F.);
#86576=ORIENTED_EDGE('',*,*,#57786,.F.);
#86577=ORIENTED_EDGE('',*,*,#57789,.F.);
#86578=ORIENTED_EDGE('',*,*,#57792,.F.);
#86579=ORIENTED_EDGE('',*,*,#57818,.F.);
#86580=ORIENTED_EDGE('',*,*,#57810,.T.);
#86581=ORIENTED_EDGE('',*,*,#57796,.T.);
#86582=ORIENTED_EDGE('',*,*,#57816,.T.);
#86583=ORIENTED_EDGE('',*,*,#57819,.T.);
#86584=ORIENTED_EDGE('',*,*,#57820,.F.);
#86585=ORIENTED_EDGE('',*,*,#57791,.T.);
#86586=ORIENTED_EDGE('',*,*,#57811,.T.);
#86587=ORIENTED_EDGE('',*,*,#57819,.F.);
#86588=ORIENTED_EDGE('',*,*,#57818,.T.);
#86589=ORIENTED_EDGE('',*,*,#57821,.F.);
#86590=ORIENTED_EDGE('',*,*,#57822,.T.);
#86591=ORIENTED_EDGE('',*,*,#57752,.T.);
#86592=ORIENTED_EDGE('',*,*,#57749,.T.);
#86593=ORIENTED_EDGE('',*,*,#57823,.T.);
#86594=ORIENTED_EDGE('',*,*,#57824,.F.);
#86595=ORIENTED_EDGE('',*,*,#57825,.F.);
#86596=ORIENTED_EDGE('',*,*,#57826,.F.);
#86597=ORIENTED_EDGE('',*,*,#57746,.F.);
#86598=ORIENTED_EDGE('',*,*,#57743,.F.);
#86599=ORIENTED_EDGE('',*,*,#57740,.F.);
#86600=ORIENTED_EDGE('',*,*,#57737,.F.);
#86601=ORIENTED_EDGE('',*,*,#57734,.F.);
#86602=ORIENTED_EDGE('',*,*,#57731,.F.);
#86603=ORIENTED_EDGE('',*,*,#57728,.F.);
#86604=ORIENTED_EDGE('',*,*,#57725,.F.);
#86605=ORIENTED_EDGE('',*,*,#57722,.F.);
#86606=ORIENTED_EDGE('',*,*,#57719,.F.);
#86607=ORIENTED_EDGE('',*,*,#57827,.F.);
#86608=ORIENTED_EDGE('',*,*,#57828,.T.);
#86609=ORIENTED_EDGE('',*,*,#57777,.T.);
#86610=ORIENTED_EDGE('',*,*,#57774,.T.);
#86611=ORIENTED_EDGE('',*,*,#57771,.T.);
#86612=ORIENTED_EDGE('',*,*,#57768,.T.);
#86613=ORIENTED_EDGE('',*,*,#57765,.T.);
#86614=ORIENTED_EDGE('',*,*,#57762,.T.);
#86615=ORIENTED_EDGE('',*,*,#57759,.T.);
#86616=ORIENTED_EDGE('',*,*,#57756,.T.);
#86617=ORIENTED_EDGE('',*,*,#57753,.T.);
#86618=ORIENTED_EDGE('',*,*,#57822,.F.);
#86619=ORIENTED_EDGE('',*,*,#57775,.T.);
#86620=ORIENTED_EDGE('',*,*,#57828,.F.);
#86621=ORIENTED_EDGE('',*,*,#57829,.F.);
#86622=ORIENTED_EDGE('',*,*,#57830,.T.);
#86623=ORIENTED_EDGE('',*,*,#57823,.F.);
#86624=ORIENTED_EDGE('',*,*,#57748,.F.);
#86625=ORIENTED_EDGE('',*,*,#57751,.F.);
#86626=ORIENTED_EDGE('',*,*,#57755,.F.);
#86627=ORIENTED_EDGE('',*,*,#57758,.F.);
#86628=ORIENTED_EDGE('',*,*,#57761,.F.);
#86629=ORIENTED_EDGE('',*,*,#57764,.F.);
#86630=ORIENTED_EDGE('',*,*,#57767,.F.);
#86631=ORIENTED_EDGE('',*,*,#57770,.F.);
#86632=ORIENTED_EDGE('',*,*,#57773,.F.);
#86633=ORIENTED_EDGE('',*,*,#57776,.F.);
#86634=ORIENTED_EDGE('',*,*,#57830,.F.);
#86635=ORIENTED_EDGE('',*,*,#57831,.F.);
#86636=ORIENTED_EDGE('',*,*,#57717,.F.);
#86637=ORIENTED_EDGE('',*,*,#57721,.F.);
#86638=ORIENTED_EDGE('',*,*,#57724,.F.);
#86639=ORIENTED_EDGE('',*,*,#57727,.F.);
#86640=ORIENTED_EDGE('',*,*,#57730,.F.);
#86641=ORIENTED_EDGE('',*,*,#57733,.F.);
#86642=ORIENTED_EDGE('',*,*,#57736,.F.);
#86643=ORIENTED_EDGE('',*,*,#57739,.F.);
#86644=ORIENTED_EDGE('',*,*,#57742,.F.);
#86645=ORIENTED_EDGE('',*,*,#57745,.F.);
#86646=ORIENTED_EDGE('',*,*,#57832,.F.);
#86647=ORIENTED_EDGE('',*,*,#57833,.F.);
#86648=ORIENTED_EDGE('',*,*,#57834,.F.);
#86649=ORIENTED_EDGE('',*,*,#57835,.F.);
#86650=ORIENTED_EDGE('',*,*,#57836,.T.);
#86651=ORIENTED_EDGE('',*,*,#57837,.F.);
#86652=ORIENTED_EDGE('',*,*,#57836,.F.);
#86653=ORIENTED_EDGE('',*,*,#57838,.F.);
#86654=ORIENTED_EDGE('',*,*,#57839,.T.);
#86655=ORIENTED_EDGE('',*,*,#57820,.T.);
#86656=ORIENTED_EDGE('',*,*,#57839,.F.);
#86657=ORIENTED_EDGE('',*,*,#57744,.T.);
#86658=ORIENTED_EDGE('',*,*,#57826,.T.);
#86659=ORIENTED_EDGE('',*,*,#57840,.F.);
#86660=ORIENTED_EDGE('',*,*,#57832,.T.);
#86661=ORIENTED_EDGE('',*,*,#57834,.T.);
#86662=ORIENTED_EDGE('',*,*,#57835,.T.);
#86663=ORIENTED_EDGE('',*,*,#57841,.T.);
#86664=ORIENTED_EDGE('',*,*,#57824,.T.);
#86665=ORIENTED_EDGE('',*,*,#57842,.T.);
#86666=ORIENTED_EDGE('',*,*,#57821,.T.);
#86667=ORIENTED_EDGE('',*,*,#57841,.F.);
#86668=ORIENTED_EDGE('',*,*,#57843,.F.);
#86669=ORIENTED_EDGE('',*,*,#57844,.T.);
#86670=ORIENTED_EDGE('',*,*,#57845,.T.);
#86671=ORIENTED_EDGE('',*,*,#57844,.F.);
#86672=ORIENTED_EDGE('',*,*,#57846,.F.);
#86673=ORIENTED_EDGE('',*,*,#57847,.T.);
#86674=ORIENTED_EDGE('',*,*,#57843,.T.);
#86675=ORIENTED_EDGE('',*,*,#57847,.F.);
#86676=ORIENTED_EDGE('',*,*,#57848,.F.);
#86677=ORIENTED_EDGE('',*,*,#57849,.T.);
#86678=ORIENTED_EDGE('',*,*,#57846,.T.);
#86679=ORIENTED_EDGE('',*,*,#57849,.F.);
#86680=ORIENTED_EDGE('',*,*,#57837,.T.);
#86681=ORIENTED_EDGE('',*,*,#57845,.F.);
#86682=ORIENTED_EDGE('',*,*,#57825,.T.);
#86683=ORIENTED_EDGE('',*,*,#57842,.F.);
#86684=ORIENTED_EDGE('',*,*,#57833,.T.);
#86685=ORIENTED_EDGE('',*,*,#57840,.T.);
#86686=ORIENTED_EDGE('',*,*,#57827,.T.);
#86687=ORIENTED_EDGE('',*,*,#57718,.F.);
#86688=ORIENTED_EDGE('',*,*,#57831,.T.);
#86689=ORIENTED_EDGE('',*,*,#57829,.T.);
#86690=ORIENTED_EDGE('',*,*,#57838,.T.);
#86691=ORIENTED_EDGE('',*,*,#57812,.T.);
#86692=ORIENTED_EDGE('',*,*,#57780,.T.);
#86693=ORIENTED_EDGE('',*,*,#57817,.T.);
#86694=ORIENTED_EDGE('',*,*,#57814,.T.);
#86695=ORIENTED_EDGE('',*,*,#57848,.T.);
#88751=CYLINDRICAL_SURFACE('',#105364,3.442);
#88752=CYLINDRICAL_SURFACE('',#105366,3.442);
#88753=CYLINDRICAL_SURFACE('',#105367,3.442);
#88754=CYLINDRICAL_SURFACE('',#105368,3.442);
#88755=CYLINDRICAL_SURFACE('',#105369,3.442);
#88756=CYLINDRICAL_SURFACE('',#105370,3.442);
#88757=CYLINDRICAL_SURFACE('',#105371,3.442);
#88758=CYLINDRICAL_SURFACE('',#105372,3.442);
#88759=CYLINDRICAL_SURFACE('',#105373,3.442);
#88760=CYLINDRICAL_SURFACE('',#105374,3.442);
#88761=CYLINDRICAL_SURFACE('',#105375,2.872);
#88762=CYLINDRICAL_SURFACE('',#105377,2.872);
#88763=CYLINDRICAL_SURFACE('',#105379,2.872);
#88764=CYLINDRICAL_SURFACE('',#105380,2.872);
#88765=CYLINDRICAL_SURFACE('',#105381,2.872);
#88766=CYLINDRICAL_SURFACE('',#105382,2.872);
#88767=CYLINDRICAL_SURFACE('',#105383,2.872);
#88768=CYLINDRICAL_SURFACE('',#105384,2.872);
#88769=CYLINDRICAL_SURFACE('',#105385,2.872);
#88770=CYLINDRICAL_SURFACE('',#105386,2.872);
#88771=CYLINDRICAL_SURFACE('',#105387,2.942);
#88772=CYLINDRICAL_SURFACE('',#105389,2.942);
#88773=CYLINDRICAL_SURFACE('',#105390,2.942);
#88774=CYLINDRICAL_SURFACE('',#105391,2.942);
#88775=CYLINDRICAL_SURFACE('',#105392,2.942);
#88776=CYLINDRICAL_SURFACE('',#105393,2.37175);
#88777=CYLINDRICAL_SURFACE('',#105395,2.37175);
#88778=CYLINDRICAL_SURFACE('',#105396,2.37175);
#88779=CYLINDRICAL_SURFACE('',#105397,2.37175);
#88780=CYLINDRICAL_SURFACE('',#105398,2.37175);
#88781=CYLINDRICAL_SURFACE('',#105399,2.37175);
#88782=CYLINDRICAL_SURFACE('',#105404,2.942);
#88783=CYLINDRICAL_SURFACE('',#105408,2.872);
#88784=CYLINDRICAL_SURFACE('',#105414,1.4);
#88785=CYLINDRICAL_SURFACE('',#105416,3.442);
#88786=CYLINDRICAL_SURFACE('',#105418,3.);
#88787=CYLINDRICAL_SURFACE('',#105420,2.1);
#88788=CYLINDRICAL_SURFACE('',#105425,1.);
#94494=ADVANCED_FACE('',(#12030),#88751,.T.);
#94495=ADVANCED_FACE('',(#12031),#88752,.T.);
#94496=ADVANCED_FACE('',(#12032),#88753,.T.);
#94497=ADVANCED_FACE('',(#12033),#88754,.T.);
#94498=ADVANCED_FACE('',(#12034),#88755,.T.);
#94499=ADVANCED_FACE('',(#12035),#88756,.T.);
#94500=ADVANCED_FACE('',(#12036),#88757,.T.);
#94501=ADVANCED_FACE('',(#12037),#88758,.T.);
#94502=ADVANCED_FACE('',(#12038),#88759,.T.);
#94503=ADVANCED_FACE('',(#12039),#88760,.T.);
#94504=ADVANCED_FACE('',(#12040),#88761,.T.);
#94505=ADVANCED_FACE('',(#12041),#88762,.T.);
#94506=ADVANCED_FACE('',(#12042),#88763,.T.);
#94507=ADVANCED_FACE('',(#12043),#88764,.T.);
#94508=ADVANCED_FACE('',(#12044),#88765,.T.);
#94509=ADVANCED_FACE('',(#12045),#88766,.T.);
#94510=ADVANCED_FACE('',(#12046),#88767,.T.);
#94511=ADVANCED_FACE('',(#12047),#88768,.T.);
#94512=ADVANCED_FACE('',(#12048),#88769,.T.);
#94513=ADVANCED_FACE('',(#12049),#88770,.T.);
#94514=ADVANCED_FACE('',(#12050),#88771,.T.);
#94515=ADVANCED_FACE('',(#12051),#88772,.T.);
#94516=ADVANCED_FACE('',(#12052),#88773,.T.);
#94517=ADVANCED_FACE('',(#12053),#88774,.T.);
#94518=ADVANCED_FACE('',(#12054),#88775,.T.);
#94519=ADVANCED_FACE('',(#12055),#88776,.T.);
#94520=ADVANCED_FACE('',(#12056),#88777,.T.);
#94521=ADVANCED_FACE('',(#12057),#88778,.T.);
#94522=ADVANCED_FACE('',(#12058),#88779,.T.);
#94523=ADVANCED_FACE('',(#12059),#88780,.T.);
#94524=ADVANCED_FACE('',(#12060),#6345,.F.);
#94525=ADVANCED_FACE('',(#12061),#88781,.T.);
#94526=ADVANCED_FACE('',(#12062),#6346,.F.);
#94527=ADVANCED_FACE('',(#12063,#5260),#6128,.F.);
#94528=ADVANCED_FACE('',(#12064),#88782,.T.);
#94529=ADVANCED_FACE('',(#12065),#6129,.F.);
#94530=ADVANCED_FACE('',(#12066),#6347,.F.);
#94531=ADVANCED_FACE('',(#12067),#88783,.T.);
#94532=ADVANCED_FACE('',(#12068),#6348,.F.);
#94533=ADVANCED_FACE('',(#12069),#5107,.T.);
#94534=ADVANCED_FACE('',(#12070),#88784,.T.);
#94535=ADVANCED_FACE('',(#12071),#88785,.T.);
#94536=ADVANCED_FACE('',(#12072),#88786,.T.);
#94537=ADVANCED_FACE('',(#12073),#88787,.F.);
#94538=ADVANCED_FACE('',(#12074),#5108,.F.);
#94539=ADVANCED_FACE('',(#12075),#88788,.F.);
#94540=ADVANCED_FACE('',(#12076,#5261),#6130,.F.);
#94541=ADVANCED_FACE('',(#12077),#6131,.F.);
#94542=ADVANCED_FACE('',(#12078,#5262),#6132,.F.);
#94543=ADVANCED_FACE('',(#12079,#5263),#6133,.F.);
#94668=CLOSED_SHELL('',(#94494,#94495,#94496,#94497,#94498,#94499,#94500,
#94501,#94502,#94503,#94504,#94505,#94506,#94507,#94508,#94509,#94510,#94511,
#94512,#94513,#94514,#94515,#94516,#94517,#94518,#94519,#94520,#94521,#94522,
#94523,#94524,#94525,#94526,#94527,#94528,#94529,#94530,#94531,#94532,#94533,
#94534,#94535,#94536,#94537,#94538,#94539,#94540,#94541,#94542,#94543));
#105363=AXIS2_PLACEMENT_3D('',#454965,#130150,#130151);
#105364=AXIS2_PLACEMENT_3D('',#454966,#130152,#130153);
#105365=AXIS2_PLACEMENT_3D('',#454982,#130155,#130156);
#105366=AXIS2_PLACEMENT_3D('',#454990,#130157,#130158);
#105367=AXIS2_PLACEMENT_3D('',#455038,#130160,#130161);
#105368=AXIS2_PLACEMENT_3D('',#455086,#130163,#130164);
#105369=AXIS2_PLACEMENT_3D('',#455140,#130166,#130167);
#105370=AXIS2_PLACEMENT_3D('',#455188,#130169,#130170);
#105371=AXIS2_PLACEMENT_3D('',#455236,#130172,#130173);
#105372=AXIS2_PLACEMENT_3D('',#455290,#130175,#130176);
#105373=AXIS2_PLACEMENT_3D('',#455338,#130178,#130179);
#105374=AXIS2_PLACEMENT_3D('',#455386,#130181,#130182);
#105375=AXIS2_PLACEMENT_3D('',#455434,#130184,#130185);
#105376=AXIS2_PLACEMENT_3D('',#455444,#130187,#130188);
#105377=AXIS2_PLACEMENT_3D('',#455445,#130189,#130190);
#105378=AXIS2_PLACEMENT_3D('',#455460,#130192,#130193);
#105379=AXIS2_PLACEMENT_3D('',#455471,#130194,#130195);
#105380=AXIS2_PLACEMENT_3D('',#455495,#130197,#130198);
#105381=AXIS2_PLACEMENT_3D('',#455519,#130200,#130201);
#105382=AXIS2_PLACEMENT_3D('',#455544,#130203,#130204);
#105383=AXIS2_PLACEMENT_3D('',#455569,#130206,#130207);
#105384=AXIS2_PLACEMENT_3D('',#455593,#130209,#130210);
#105385=AXIS2_PLACEMENT_3D('',#455618,#130212,#130213);
#105386=AXIS2_PLACEMENT_3D('',#455643,#130215,#130216);
#105387=AXIS2_PLACEMENT_3D('',#455667,#130218,#130219);
#105388=AXIS2_PLACEMENT_3D('',#455683,#130221,#130222);
#105389=AXIS2_PLACEMENT_3D('',#455691,#130223,#130224);
#105390=AXIS2_PLACEMENT_3D('',#455739,#130226,#130227);
#105391=AXIS2_PLACEMENT_3D('',#455787,#130229,#130230);
#105392=AXIS2_PLACEMENT_3D('',#455841,#130232,#130233);
#105393=AXIS2_PLACEMENT_3D('',#455889,#130235,#130236);
#105394=AXIS2_PLACEMENT_3D('',#455901,#130238,#130239);
#105395=AXIS2_PLACEMENT_3D('',#455906,#130240,#130241);
#105396=AXIS2_PLACEMENT_3D('',#455931,#130243,#130244);
#105397=AXIS2_PLACEMENT_3D('',#455956,#130246,#130247);
#105398=AXIS2_PLACEMENT_3D('',#455981,#130249,#130250);
#105399=AXIS2_PLACEMENT_3D('',#456365,#130252,#130253);
#105400=AXIS2_PLACEMENT_3D('',#456367,#130254,#130255);
#105401=AXIS2_PLACEMENT_3D('',#456723,#130256,#130257);
#105402=AXIS2_PLACEMENT_3D('',#456724,#130258,#130259);
#105403=AXIS2_PLACEMENT_3D('',#456726,#130260,#130261);
#105404=AXIS2_PLACEMENT_3D('',#456727,#130262,#130263);
#105405=AXIS2_PLACEMENT_3D('',#456728,#130264,#130265);
#105406=AXIS2_PLACEMENT_3D('',#456731,#130266,#130267);
#105407=AXIS2_PLACEMENT_3D('',#456774,#130268,#130269);
#105408=AXIS2_PLACEMENT_3D('',#457228,#130270,#130271);
#105409=AXIS2_PLACEMENT_3D('',#457230,#130272,#130273);
#105410=AXIS2_PLACEMENT_3D('',#457682,#130274,#130275);
#105411=AXIS2_PLACEMENT_3D('',#457685,#130276,#130277);
#105412=AXIS2_PLACEMENT_3D('',#457686,#130278,#130279);
#105413=AXIS2_PLACEMENT_3D('',#457689,#130281,#130282);
#105414=AXIS2_PLACEMENT_3D('',#457690,#130283,#130284);
#105415=AXIS2_PLACEMENT_3D('',#457692,#130285,#130286);
#105416=AXIS2_PLACEMENT_3D('',#457694,#130288,#130289);
#105417=AXIS2_PLACEMENT_3D('',#457695,#130290,#130291);
#105418=AXIS2_PLACEMENT_3D('',#457696,#130292,#130293);
#105419=AXIS2_PLACEMENT_3D('',#457698,#130295,#130296);
#105420=AXIS2_PLACEMENT_3D('',#457699,#130297,#130298);
#105421=AXIS2_PLACEMENT_3D('',#457701,#130299,#130300);
#105422=AXIS2_PLACEMENT_3D('',#457704,#130302,#130303);
#105423=AXIS2_PLACEMENT_3D('',#457705,#130304,#130305);
#105424=AXIS2_PLACEMENT_3D('',#457707,#130306,#130307);
#105425=AXIS2_PLACEMENT_3D('',#457709,#130309,#130310);
#105426=AXIS2_PLACEMENT_3D('',#457711,#130311,#130312);
#105427=AXIS2_PLACEMENT_3D('',#457713,#130314,#130315);
#105428=AXIS2_PLACEMENT_3D('',#457714,#130316,#130317);
#105429=AXIS2_PLACEMENT_3D('',#457715,#130318,#130319);
#105430=AXIS2_PLACEMENT_3D('',#457716,#130320,#130321);
#130150=DIRECTION('axis',(0.,0.,1.));
#130151=DIRECTION('refdir',(1.,0.,0.));
#130152=DIRECTION('center_axis',(0.,1.,0.));
#130153=DIRECTION('ref_axis',(0.,0.,1.));
#130154=DIRECTION('',(0.,-1.,0.));
#130155=DIRECTION('center_axis',(0.,-1.,0.));
#130156=DIRECTION('ref_axis',(0.,0.,1.));
#130157=DIRECTION('center_axis',(0.,1.,0.));
#130158=DIRECTION('ref_axis',(0.,0.,1.));
#130159=DIRECTION('',(0.,-1.,0.));
#130160=DIRECTION('center_axis',(0.,1.,0.));
#130161=DIRECTION('ref_axis',(0.,0.,1.));
#130162=DIRECTION('',(0.,-1.,0.));
#130163=DIRECTION('center_axis',(0.,1.,0.));
#130164=DIRECTION('ref_axis',(0.,0.,1.));
#130165=DIRECTION('',(0.,-1.,0.));
#130166=DIRECTION('center_axis',(0.,1.,0.));
#130167=DIRECTION('ref_axis',(0.,0.,1.));
#130168=DIRECTION('',(0.,-1.,0.));
#130169=DIRECTION('center_axis',(0.,1.,0.));
#130170=DIRECTION('ref_axis',(0.,0.,1.));
#130171=DIRECTION('',(0.,-1.,0.));
#130172=DIRECTION('center_axis',(0.,1.,0.));
#130173=DIRECTION('ref_axis',(0.,0.,1.));
#130174=DIRECTION('',(0.,-1.,0.));
#130175=DIRECTION('center_axis',(0.,1.,0.));
#130176=DIRECTION('ref_axis',(0.,0.,1.));
#130177=DIRECTION('',(0.,-1.,0.));
#130178=DIRECTION('center_axis',(0.,1.,0.));
#130179=DIRECTION('ref_axis',(0.,0.,1.));
#130180=DIRECTION('',(0.,-1.,0.));
#130181=DIRECTION('center_axis',(0.,1.,0.));
#130182=DIRECTION('ref_axis',(0.,0.,1.));
#130183=DIRECTION('',(0.,-1.,0.));
#130184=DIRECTION('center_axis',(0.,1.,0.));
#130185=DIRECTION('ref_axis',(5.13873024532413E-14,0.,1.));
#130186=DIRECTION('',(0.,1.,0.));
#130187=DIRECTION('center_axis',(0.,1.,0.));
#130188=DIRECTION('ref_axis',(5.13873024532413E-14,0.,1.));
#130189=DIRECTION('center_axis',(0.,1.,0.));
#130190=DIRECTION('ref_axis',(5.13873024532413E-14,0.,1.));
#130191=DIRECTION('',(0.,1.,0.));
#130192=DIRECTION('center_axis',(0.,1.,0.));
#130193=DIRECTION('ref_axis',(5.13873024532413E-14,0.,1.));
#130194=DIRECTION('center_axis',(0.,1.,0.));
#130195=DIRECTION('ref_axis',(5.13873024532413E-14,0.,1.));
#130196=DIRECTION('',(0.,1.,0.));
#130197=DIRECTION('center_axis',(0.,1.,0.));
#130198=DIRECTION('ref_axis',(5.13873024532413E-14,0.,1.));
#130199=DIRECTION('',(0.,1.,0.));
#130200=DIRECTION('center_axis',(0.,1.,0.));
#130201=DIRECTION('ref_axis',(5.13873024532413E-14,0.,1.));
#130202=DIRECTION('',(0.,1.,0.));
#130203=DIRECTION('center_axis',(0.,1.,0.));
#130204=DIRECTION('ref_axis',(5.13873024532413E-14,0.,1.));
#130205=DIRECTION('',(0.,1.,0.));
#130206=DIRECTION('center_axis',(0.,1.,0.));
#130207=DIRECTION('ref_axis',(5.13873024532413E-14,0.,1.));
#130208=DIRECTION('',(0.,1.,0.));
#130209=DIRECTION('center_axis',(0.,1.,0.));
#130210=DIRECTION('ref_axis',(5.13873024532413E-14,0.,1.));
#130211=DIRECTION('',(0.,1.,0.));
#130212=DIRECTION('center_axis',(0.,1.,0.));
#130213=DIRECTION('ref_axis',(5.13873024532413E-14,0.,1.));
#130214=DIRECTION('',(0.,1.,0.));
#130215=DIRECTION('center_axis',(0.,1.,0.));
#130216=DIRECTION('ref_axis',(5.13873024532413E-14,0.,1.));
#130217=DIRECTION('',(0.,1.,0.));
#130218=DIRECTION('center_axis',(0.,1.,0.));
#130219=DIRECTION('ref_axis',(0.,0.,1.));
#130220=DIRECTION('',(0.,-1.,0.));
#130221=DIRECTION('center_axis',(0.,-1.,0.));
#130222=DIRECTION('ref_axis',(0.,0.,1.));
#130223=DIRECTION('center_axis',(0.,1.,0.));
#130224=DIRECTION('ref_axis',(0.,0.,1.));
#130225=DIRECTION('',(0.,-1.,0.));
#130226=DIRECTION('center_axis',(0.,1.,0.));
#130227=DIRECTION('ref_axis',(0.,0.,1.));
#130228=DIRECTION('',(0.,-1.,0.));
#130229=DIRECTION('center_axis',(0.,1.,0.));
#130230=DIRECTION('ref_axis',(0.,0.,1.));
#130231=DIRECTION('',(0.,-1.,0.));
#130232=DIRECTION('center_axis',(0.,1.,0.));
#130233=DIRECTION('ref_axis',(0.,0.,1.));
#130234=DIRECTION('',(0.,-1.,0.));
#130235=DIRECTION('center_axis',(0.,1.,0.));
#130236=DIRECTION('ref_axis',(4.71072660257168E-15,0.,1.));
#130237=DIRECTION('',(0.,1.,0.));
#130238=DIRECTION('center_axis',(0.,1.,0.));
#130239=DIRECTION('ref_axis',(4.71072660257168E-15,0.,1.));
#130240=DIRECTION('center_axis',(0.,1.,0.));
#130241=DIRECTION('ref_axis',(4.71072660257168E-15,0.,1.));
#130242=DIRECTION('',(0.,1.,0.));
#130243=DIRECTION('center_axis',(0.,1.,0.));
#130244=DIRECTION('ref_axis',(4.71072660257168E-15,0.,1.));
#130245=DIRECTION('',(0.,1.,0.));
#130246=DIRECTION('center_axis',(0.,1.,0.));
#130247=DIRECTION('ref_axis',(4.71072660257168E-15,0.,1.));
#130248=DIRECTION('',(0.,1.,0.));
#130249=DIRECTION('center_axis',(0.,1.,0.));
#130250=DIRECTION('ref_axis',(4.71072660257168E-15,0.,1.));
#130251=DIRECTION('',(0.,1.,0.));
#130252=DIRECTION('center_axis',(0.,1.,0.));
#130253=DIRECTION('ref_axis',(0.457752838279926,0.,0.889079489723316));
#130254=DIRECTION('center_axis',(0.,-1.,0.));
#130255=DIRECTION('ref_axis',(4.71072660257168E-15,0.,1.));
#130256=DIRECTION('center_axis',(0.,-1.,0.));
#130257=DIRECTION('ref_axis',(0.,0.,-1.));
#130258=DIRECTION('center_axis',(0.,1.,0.));
#130259=DIRECTION('ref_axis',(0.,0.,1.));
#130260=DIRECTION('center_axis',(0.,1.,0.));
#130261=DIRECTION('ref_axis',(0.,0.,1.));
#130262=DIRECTION('center_axis',(0.,1.,0.));
#130263=DIRECTION('ref_axis',(0.,0.,1.));
#130264=DIRECTION('center_axis',(0.,1.,0.));
#130265=DIRECTION('ref_axis',(0.,0.,1.));
#130266=DIRECTION('center_axis',(0.,1.,0.));
#130267=DIRECTION('ref_axis',(0.,0.,1.));
#130268=DIRECTION('center_axis',(0.,1.,0.));
#130269=DIRECTION('ref_axis',(0.,0.,1.));
#130270=DIRECTION('center_axis',(0.,1.,0.));
#130271=DIRECTION('ref_axis',(5.13873024532413E-14,0.,1.));
#130272=DIRECTION('center_axis',(0.,-1.,0.));
#130273=DIRECTION('ref_axis',(5.13873024532413E-14,0.,1.));
#130274=DIRECTION('center_axis',(0.,-1.,0.));
#130275=DIRECTION('ref_axis',(0.,0.,-1.));
#130276=DIRECTION('center_axis',(0.,-1.,0.));
#130277=DIRECTION('ref_axis',(0.,0.,-1.));
#130278=DIRECTION('center_axis',(0.,-1.,0.));
#130279=DIRECTION('ref_axis',(0.,0.,-1.));
#130280=DIRECTION('',(8.65956056235495E-17,0.707106781186546,-0.707106781186549));
#130281=DIRECTION('center_axis',(0.,1.,0.));
#130282=DIRECTION('ref_axis',(0.,0.,-1.));
#130283=DIRECTION('center_axis',(0.,1.,0.));
#130284=DIRECTION('ref_axis',(0.,0.,1.));
#130285=DIRECTION('center_axis',(0.,1.,0.));
#130286=DIRECTION('ref_axis',(0.,0.,1.));
#130287=DIRECTION('',(0.,-1.,0.));
#130288=DIRECTION('center_axis',(0.,1.,0.));
#130289=DIRECTION('ref_axis',(0.,0.,1.));
#130290=DIRECTION('center_axis',(0.,1.,0.));
#130291=DIRECTION('ref_axis',(0.,0.,1.));
#130292=DIRECTION('center_axis',(0.,1.,0.));
#130293=DIRECTION('ref_axis',(0.,0.,1.));
#130294=DIRECTION('',(0.,-1.,0.));
#130295=DIRECTION('center_axis',(0.,1.,0.));
#130296=DIRECTION('ref_axis',(0.,0.,1.));
#130297=DIRECTION('center_axis',(0.,1.,0.));
#130298=DIRECTION('ref_axis',(0.,0.,1.));
#130299=DIRECTION('center_axis',(0.,1.,0.));
#130300=DIRECTION('ref_axis',(0.,0.,1.));
#130301=DIRECTION('',(0.,1.,0.));
#130302=DIRECTION('center_axis',(0.,1.,0.));
#130303=DIRECTION('ref_axis',(0.,0.,1.));
#130304=DIRECTION('center_axis',(0.,1.,0.));
#130305=DIRECTION('ref_axis',(0.,0.,1.));
#130306=DIRECTION('center_axis',(0.,1.,0.));
#130307=DIRECTION('ref_axis',(0.,0.,1.));
#130308=DIRECTION('',(-8.65956056235495E-17,0.707106781186546,-0.707106781186549));
#130309=DIRECTION('center_axis',(0.,1.,0.));
#130310=DIRECTION('ref_axis',(0.,0.,1.));
#130311=DIRECTION('center_axis',(0.,1.,0.));
#130312=DIRECTION('ref_axis',(0.,0.,1.));
#130313=DIRECTION('',(0.,1.,0.));
#130314=DIRECTION('center_axis',(0.,-1.,0.));
#130315=DIRECTION('ref_axis',(0.,0.,-1.));
#130316=DIRECTION('center_axis',(0.,-1.,0.));
#130317=DIRECTION('ref_axis',(0.,0.,-1.));
#130318=DIRECTION('center_axis',(0.,1.,0.));
#130319=DIRECTION('ref_axis',(0.,0.,1.));
#130320=DIRECTION('center_axis',(0.,1.,0.));
#130321=DIRECTION('ref_axis',(0.,0.,1.));
#454965=CARTESIAN_POINT('',(0.,0.,0.));
#454966=CARTESIAN_POINT('Origin',(0.,0.,0.));
#454967=CARTESIAN_POINT('',(0.00238312071812623,7.42232045465689,-3.44573997435601));
#454968=CARTESIAN_POINT('',(0.00358895744866569,7.2776795453431,-3.44504374594936));
#454969=CARTESIAN_POINT('',(-4.21523428266519E-16,0.,-3.442));
#454970=CARTESIAN_POINT('',(3.09271722244255,7.1,1.51078263890185));
#454971=CARTESIAN_POINT('Ctrl Pts',(0.00238312071812623,7.42232045465689,
-3.44573997435601));
#454972=CARTESIAN_POINT('Ctrl Pts',(0.134189165843592,7.41620645307186,
-3.44671132434039));
#454973=CARTESIAN_POINT('Ctrl Pts',(0.265886689822806,7.41009245148682,
-3.43980123267601));
#454974=CARTESIAN_POINT('Ctrl Pts',(0.396625140499449,7.40397844990179,
-3.42466879815526));
#454975=CARTESIAN_POINT('Ctrl Pts',(1.52472351508465,7.35122277462346,-3.29409608065693));
#454976=CARTESIAN_POINT('Ctrl Pts',(2.58141517031108,7.29846709934514,-2.55133811387537));
#454977=CARTESIAN_POINT('Ctrl Pts',(3.08712931628112,7.24571142406682,-1.5341055545258));
#454978=CARTESIAN_POINT('Ctrl Pts',(3.55272426880691,7.19714094937788,-0.597571844815975));
#454979=CARTESIAN_POINT('Ctrl Pts',(3.55129415105041,7.14857047468894,0.571614765840351));
#454980=CARTESIAN_POINT('Ctrl Pts',(3.09699338763787,7.1,1.51441171489142));
#454981=CARTESIAN_POINT('',(3.09271722244257,7.1,-1.51078263890182));
#454982=CARTESIAN_POINT('Origin',(0.,7.1,0.));
#454983=CARTESIAN_POINT('Ctrl Pts',(3.09271722244257,7.1,-1.51078263890182));
#454984=CARTESIAN_POINT('Ctrl Pts',(2.59193253573628,7.15275567527832,-2.53593700951191));
#454985=CARTESIAN_POINT('Ctrl Pts',(1.54584605382252,7.20551135055665,-3.28388805779909));
#454986=CARTESIAN_POINT('Ctrl Pts',(0.420315138273282,7.25826702583497,
-3.42154258483277));
#454987=CARTESIAN_POINT('Ctrl Pts',(0.282261170683799,7.26473786567101,
-3.43842684216513));
#454988=CARTESIAN_POINT('Ctrl Pts',(0.143011987085937,7.27120870550706,
-3.44612938419434));
#454989=CARTESIAN_POINT('Ctrl Pts',(0.00358895744866569,7.2776795453431,
-3.44504374594936));
#454990=CARTESIAN_POINT('Origin',(0.,0.,0.));
#454991=CARTESIAN_POINT('',(0.00119116194521041,8.42232045465689,-3.43683718515566));
#454992=CARTESIAN_POINT('',(0.00109290156775514,8.2776795453431,-3.43675318504777));
#454993=CARTESIAN_POINT('',(-4.21523428266519E-16,0.,-3.442));
#454994=CARTESIAN_POINT('Ctrl Pts',(0.00119116194521041,8.42232045465689,
-3.43683718515566));
#454995=CARTESIAN_POINT('Ctrl Pts',(0.49847441043924,8.39940717140846,-3.43838762583654));
#454996=CARTESIAN_POINT('Ctrl Pts',(0.995157371276851,8.37649388816004,
-3.33748454788281));
#454997=CARTESIAN_POINT('Ctrl Pts',(1.44316539496645,8.35358060491161,-3.1309843016151));
#454998=CARTESIAN_POINT('Ctrl Pts',(2.47466164819217,8.30082492963329,-2.65553694564786));
#454999=CARTESIAN_POINT('Ctrl Pts',(3.24812854171467,8.24806925435496,-1.62031136862869));
#455000=CARTESIAN_POINT('Ctrl Pts',(3.41165377002092,8.19531357907664,-0.496342238358058));
#455001=CARTESIAN_POINT('Ctrl Pts',(3.57517899832716,8.14255790379832,0.627626891912579));
#455002=CARTESIAN_POINT('Ctrl Pts',(3.12876256141716,8.08980222851999,1.84033957543469));
#455003=CARTESIAN_POINT('Ctrl Pts',(2.27548272011085,8.03704655324167,2.58998788073998));
#455004=CARTESIAN_POINT('Ctrl Pts',(1.42220287880454,7.98429087796335,3.33963618604527));
#455005=CARTESIAN_POINT('Ctrl Pts',(0.162059633101916,7.93153520268503,
3.62622011313374));
#455006=CARTESIAN_POINT('Ctrl Pts',(-0.931477912766307,7.8787795274067,
3.31935910596737));
#455007=CARTESIAN_POINT('Ctrl Pts',(-2.02501545863453,7.82602385212838,
3.01249809880101));
#455008=CARTESIAN_POINT('Ctrl Pts',(-2.95194730466835,7.77326817685005,
2.1121921573798));
#455009=CARTESIAN_POINT('Ctrl Pts',(-3.29068060623052,7.72051250157173,
1.02805540866212));
#455010=CARTESIAN_POINT('Ctrl Pts',(-3.62941390779269,7.66775682629341,
-0.0560813400555474));
#455011=CARTESIAN_POINT('Ctrl Pts',(-3.37994866488321,7.61500115101509,
-1.32404889606968));
#455012=CARTESIAN_POINT('Ctrl Pts',(-2.65546349645648,7.56224547573676,
-2.19883893996919));
#455013=CARTESIAN_POINT('Ctrl Pts',(-2.01494092437082,7.51560380204347,
-2.97224713846996));
#455014=CARTESIAN_POINT('Ctrl Pts',(-1.00312112425844,7.46896212835018,
-3.43832987012503));
#455015=CARTESIAN_POINT('Ctrl Pts',(0.00238312071812623,7.42232045465689,
-3.44573997435601));
#455016=CARTESIAN_POINT('Ctrl Pts',(0.00358895744866569,7.2776795453431,
-3.44504374594936));
#455017=CARTESIAN_POINT('Ctrl Pts',(-0.993680662435879,7.32396438078538,
-3.43727835709852));
#455018=CARTESIAN_POINT('Ctrl Pts',(-1.99984477020885,7.37024921622766,
-2.97988315053305));
#455019=CARTESIAN_POINT('Ctrl Pts',(-2.6411222941201,7.41653405166994,-2.21687640500152));
#455020=CARTESIAN_POINT('Ctrl Pts',(-3.3720534617795,7.46928972694826,-1.34719769235643));
#455021=CARTESIAN_POINT('Ctrl Pts',(-3.6289404479136,7.52204540222659,-0.080482261286085));
#455022=CARTESIAN_POINT('Ctrl Pts',(-3.29723843930749,7.57480107750491,
1.00601810569489));
#455023=CARTESIAN_POINT('Ctrl Pts',(-2.96553643070138,7.62755675278323,
2.09251847267586));
#455024=CARTESIAN_POINT('Ctrl Pts',(-2.04524542735508,7.68031242806155,
2.99880377556747));
#455025=CARTESIAN_POINT('Ctrl Pts',(-0.953932543642956,7.73306810333988,
3.31295667324589));
#455026=CARTESIAN_POINT('Ctrl Pts',(0.13738034006917,7.7858237786182,3.62710957092432));
#455027=CARTESIAN_POINT('Ctrl Pts',(1.39971510414711,7.83857945389653,3.34913006338957));
#455028=CARTESIAN_POINT('Ctrl Pts',(2.25808828818259,7.89133512917485,2.60526729131064));
#455029=CARTESIAN_POINT('Ctrl Pts',(3.11646147221806,7.94409080445317,1.86140451923172));
#455030=CARTESIAN_POINT('Ctrl Pts',(3.57087307621107,7.99684647973149,0.651658482608627));
#455031=CARTESIAN_POINT('Ctrl Pts',(3.41487509938555,8.04960215500982,-0.473400457015574));
#455032=CARTESIAN_POINT('Ctrl Pts',(3.25887712256003,8.10235783028814,-1.59845939663978));
#455033=CARTESIAN_POINT('Ctrl Pts',(2.49246956491597,8.15511350556647,-2.6388312392651));
#455034=CARTESIAN_POINT('Ctrl Pts',(1.4642134312474,8.20786918084479,-3.12119802101246));
#455035=CARTESIAN_POINT('Ctrl Pts',(1.01065758087162,8.23113930234422,-3.3339662883));
#455036=CARTESIAN_POINT('Ctrl Pts',(0.506155841458834,8.25440942384366,
-3.43816774821673));
#455037=CARTESIAN_POINT('Ctrl Pts',(0.00109290156775514,8.2776795453431,
-3.43675318504777));
#455038=CARTESIAN_POINT('Origin',(0.,0.,0.));
#455039=CARTESIAN_POINT('',(-0.00309368505836849,9.42232045465689,-3.44152090478281));
#455040=CARTESIAN_POINT('',(-0.00309581765146611,9.2776795453431,-3.4417505667627));
#455041=CARTESIAN_POINT('',(-4.21523428266519E-16,0.,-3.442));
#455042=CARTESIAN_POINT('Ctrl Pts',(-0.00309368505836849,9.42232045465689,
-3.44152090478281));
#455043=CARTESIAN_POINT('Ctrl Pts',(0.855820397317136,9.38260788974507,
-3.43381237529938));
#455044=CARTESIAN_POINT('Ctrl Pts',(1.71995527738355,9.34289532483326,-3.10781983641605));
#455045=CARTESIAN_POINT('Ctrl Pts',(2.34637752785182,9.30318275992144,-2.5259247880675));
#455046=CARTESIAN_POINT('Ctrl Pts',(3.17854057010811,9.25042708464312,-1.75291336750315));
#455047=CARTESIAN_POINT('Ctrl Pts',(3.5912009188089,9.19767140936479,-0.528298714120453));
#455048=CARTESIAN_POINT('Ctrl Pts',(3.39659380113874,9.14491573408646,0.590705393077353));
#455049=CARTESIAN_POINT('Ctrl Pts',(3.20198668346858,9.09216005880813,1.70970950027516));
#455050=CARTESIAN_POINT('Ctrl Pts',(2.40011209942749,9.03940438352981,2.72310306128807));
#455051=CARTESIAN_POINT('Ctrl Pts',(1.35583137668917,8.98664870825149,3.16978005845081));
#455052=CARTESIAN_POINT('Ctrl Pts',(0.311550653950845,8.93389303297317,
3.61645705561355));
#455053=CARTESIAN_POINT('Ctrl Pts',(-0.975136207484709,8.88113735769485,
3.49641748892612));
#455054=CARTESIAN_POINT('Ctrl Pts',(-1.91876999931101,8.82838168241653,
2.86428111708987));
#455055=CARTESIAN_POINT('Ctrl Pts',(-2.86240379113731,8.7756260071382,2.23214474525363));
#455056=CARTESIAN_POINT('Ctrl Pts',(-3.46298451335436,8.72287033185987,
1.08791156826856));
#455057=CARTESIAN_POINT('Ctrl Pts',(-3.44724434922051,8.67011465658155,
-0.0477797400067174));
#455058=CARTESIAN_POINT('Ctrl Pts',(-3.43150418508666,8.61735898130322,
-1.183471048282));
#455059=CARTESIAN_POINT('Ctrl Pts',(-2.79944313460191,8.56460330602491,
-2.31062048784749));
#455060=CARTESIAN_POINT('Ctrl Pts',(-1.83864980289507,8.51184763074659,
-2.91636064017258));
#455061=CARTESIAN_POINT('Ctrl Pts',(-1.29515621451355,8.48200523871669,
-3.25901069627681));
#455062=CARTESIAN_POINT('Ctrl Pts',(-0.646473404086736,8.45216284668679,
-3.43481788228595));
#455063=CARTESIAN_POINT('Ctrl Pts',(0.00119116194521041,8.42232045465689,
-3.43683718515566));
#455064=CARTESIAN_POINT('Ctrl Pts',(0.00109290156775514,8.2776795453431,
-3.43675318504777));
#455065=CARTESIAN_POINT('Ctrl Pts',(-0.638871976838291,8.30716509912199,
-3.43496079310031));
#455066=CARTESIAN_POINT('Ctrl Pts',(-1.27973788536319,8.33665065290087,
-3.26359759443701));
#455067=CARTESIAN_POINT('Ctrl Pts',(-1.81900325993667,8.36613620667976,
-2.92866660332892));
#455068=CARTESIAN_POINT('Ctrl Pts',(-2.78385910775911,8.41889188195808,
-2.32940668302862));
#455069=CARTESIAN_POINT('Ctrl Pts',(-3.42346609371094,8.4716475572364,-1.20652512155862));
#455070=CARTESIAN_POINT('Ctrl Pts',(-3.44683967457762,8.52440323251473,
-0.0709631335329957));
#455071=CARTESIAN_POINT('Ctrl Pts',(-3.4702132554443,8.57715890779305,1.06459885449263));
#455072=CARTESIAN_POINT('Ctrl Pts',(-2.87735343122583,8.62991458307138,
2.21284126907387));
#455073=CARTESIAN_POINT('Ctrl Pts',(-1.93799541836559,8.6826702583497,2.85130935660359));
#455074=CARTESIAN_POINT('Ctrl Pts',(-0.998637405505343,8.73542593362803,
3.4897774441333));
#455075=CARTESIAN_POINT('Ctrl Pts',(0.287218795996676,8.78818160890635,
3.6184712046115));
#455076=CARTESIAN_POINT('Ctrl Pts',(1.33448180904785,8.84093728418467,3.17882887749084));
#455077=CARTESIAN_POINT('Ctrl Pts',(2.38174482209902,8.89369295946299,2.73918655037018));
#455078=CARTESIAN_POINT('Ctrl Pts',(3.19041464669936,8.94644863474132,1.73120813565067));
#455079=CARTESIAN_POINT('Ctrl Pts',(3.39254330235197,8.99920431001964,0.613537900451479));
#455080=CARTESIAN_POINT('Ctrl Pts',(3.59467195800459,9.05195998529796,-0.504132334747713));
#455081=CARTESIAN_POINT('Ctrl Pts',(3.19025944470949,9.10471566057628,-1.73149439042658));
#455082=CARTESIAN_POINT('Ctrl Pts',(2.36331494236584,9.1574713358546,-2.51008553228953));
#455083=CARTESIAN_POINT('Ctrl Pts',(1.73522758526385,9.19754073901743,-3.1014471668004));
#455084=CARTESIAN_POINT('Ctrl Pts',(0.863388912503553,9.23761014218027,
-3.43392070879517));
#455085=CARTESIAN_POINT('Ctrl Pts',(-0.0030958176514661,9.2776795453431,
-3.4417505667627));
#455086=CARTESIAN_POINT('Origin',(0.,0.,0.));
#455087=CARTESIAN_POINT('',(0.00142507496518784,10.4223204546569,-3.44683866470506));
#455088=CARTESIAN_POINT('',(0.00154693548059185,10.2776795453431,-3.44670349103507));
#455089=CARTESIAN_POINT('',(-4.21523428266519E-16,0.,-3.442));
#455090=CARTESIAN_POINT('Ctrl Pts',(0.00142507496518784,10.4223204546569,
-3.44683866470506));
#455091=CARTESIAN_POINT('Ctrl Pts',(0.0823396048270201,10.41856428336,-3.44726368601611));
#455092=CARTESIAN_POINT('Ctrl Pts',(0.163226312415324,10.4148081120631,
-3.44465965322517));
#455093=CARTESIAN_POINT('Ctrl Pts',(0.243891972020051,10.4110519407662,
-3.43893878754763));
#455094=CARTESIAN_POINT('Ctrl Pts',(1.37684651744847,10.3582962654879,-3.35858884923533));
#455095=CARTESIAN_POINT('Ctrl Pts',(2.46619627771366,10.3055405902096,-2.66340033058106));
#455096=CARTESIAN_POINT('Ctrl Pts',(3.01627446688699,10.2527849149312,-1.6696920751257));
#455097=CARTESIAN_POINT('Ctrl Pts',(3.56635265606032,10.2000292396529,-0.675983819670343));
#455098=CARTESIAN_POINT('Ctrl Pts',(3.5771592741418,10.1472735643746,0.616244172586106));
#455099=CARTESIAN_POINT('Ctrl Pts',(3.04377719383542,10.0945178890963,1.61901317285293));
#455100=CARTESIAN_POINT('Ctrl Pts',(2.51039511352904,10.041762213818,2.62178217311977));
#455101=CARTESIAN_POINT('Ctrl Pts',(1.43282433483482,9.98900653853964,3.33509218139697));
#455102=CARTESIAN_POINT('Ctrl Pts',(0.301372047598186,9.93625086326132,
3.43437886338635));
#455103=CARTESIAN_POINT('Ctrl Pts',(-0.830080239638436,9.88349518798299,
3.53366554537574));
#455104=CARTESIAN_POINT('Ctrl Pts',(-2.01541403541746,9.83073951270466,
3.0189289010773));
#455105=CARTESIAN_POINT('Ctrl Pts',(-2.71528867421011,9.77798383742634,
2.12438008348235));
#455106=CARTESIAN_POINT('Ctrl Pts',(-3.41516331300278,9.72522816214802,
1.22983126588738));
#455107=CARTESIAN_POINT('Ctrl Pts',(-3.62957879480908,9.6724724868697,-0.0445297250041106));
#455108=CARTESIAN_POINT('Ctrl Pts',(-3.26097365394768,9.61971681159138,
-1.11885386515457));
#455109=CARTESIAN_POINT('Ctrl Pts',(-2.89236851308627,9.56696113631306,
-2.19317800530503));
#455110=CARTESIAN_POINT('Ctrl Pts',(-1.94074274955717,9.51420546103472,
-3.06746529471446));
#455111=CARTESIAN_POINT('Ctrl Pts',(-0.839096999886727,9.4614497857564,
-3.34390484554616));
#455112=CARTESIAN_POINT('Ctrl Pts',(-0.566730339391244,9.44840667538989,
-3.41225069747854));
#455113=CARTESIAN_POINT('Ctrl Pts',(-0.285193599698565,9.43536356502339,
-3.44405267781331));
#455114=CARTESIAN_POINT('Ctrl Pts',(-0.00309368505836849,9.42232045465689,
-3.44152090478281));
#455115=CARTESIAN_POINT('Ctrl Pts',(-0.0030958176514661,9.2776795453431,
-3.4417505667627));
#455116=CARTESIAN_POINT('Ctrl Pts',(-0.277431350576604,9.29036581745859,
-3.44422955823652));
#455117=CARTESIAN_POINT('Ctrl Pts',(-0.551230202762694,9.30305208957409,
-3.4141661739107));
#455118=CARTESIAN_POINT('Ctrl Pts',(-0.816586564771066,9.31573836168958,
-3.34947354022971));
#455119=CARTESIAN_POINT('Ctrl Pts',(-1.92006707817213,9.36849403696791,
-3.08045017825992));
#455120=CARTESIAN_POINT('Ctrl Pts',(-2.87755161358206,9.42124971224623,
-2.21258322627329));
#455121=CARTESIAN_POINT('Ctrl Pts',(-3.25337446224197,9.47400538752455,
-1.14076255284959));
#455122=CARTESIAN_POINT('Ctrl Pts',(-3.62919731090188,9.52676106280287,
-0.0689418794258828));
#455123=CARTESIAN_POINT('Ctrl Pts',(-3.42335847281178,9.5795167380812,1.2068325154349));
#455124=CARTESIAN_POINT('Ctrl Pts',(-2.72951655849602,9.63227241335952,
2.10606865285624));
#455125=CARTESIAN_POINT('Ctrl Pts',(-2.03567464418025,9.68502808863784,
3.00530479027758));
#455126=CARTESIAN_POINT('Ctrl Pts',(-0.853829653638802,9.73778376391616,
3.52800267025948));
#455127=CARTESIAN_POINT('Ctrl Pts',(0.278264995679193,9.79053943919449,
3.43632860190599));
#455128=CARTESIAN_POINT('Ctrl Pts',(1.41035964499719,9.84329511447281,3.3446545335525));
#455129=CARTESIAN_POINT('Ctrl Pts',(2.49270395309174,9.89605078975114,2.63860851686363));
#455130=CARTESIAN_POINT('Ctrl Pts',(3.03281882209306,9.94880646502946,1.63944972893749));
#455131=CARTESIAN_POINT('Ctrl Pts',(3.57293369109439,10.0015621403078,0.640290941011352));
#455132=CARTESIAN_POINT('Ctrl Pts',(3.5708191210025,10.0543178155861,-0.651980618152043));
#455133=CARTESIAN_POINT('Ctrl Pts',(3.02743720280062,10.1070734908644,-1.6493664187819));
#455134=CARTESIAN_POINT('Ctrl Pts',(2.48405528459874,10.1598291661428,-2.64675221941176));
#455135=CARTESIAN_POINT('Ctrl Pts',(1.39940601828685,10.2125848414211,-3.34925226150807));
#455136=CARTESIAN_POINT('Ctrl Pts',(0.267017438351514,10.2653405166994,
-3.43722086185585));
#455137=CARTESIAN_POINT('Ctrl Pts',(0.178732623179784,10.2694535262473,
-3.44407918925355));
#455138=CARTESIAN_POINT('Ctrl Pts',(0.0901576348521517,10.2735665357952,
-3.44720221938116));
#455139=CARTESIAN_POINT('Ctrl Pts',(0.00154693548059185,10.2776795453431,
-3.44670349103507));
#455140=CARTESIAN_POINT('Origin',(0.,0.,0.));
#455141=CARTESIAN_POINT('',(0.00190492198109293,11.4223204546569,-3.43753765796313));
#455142=CARTESIAN_POINT('',(0.00180381072558041,11.2776795453431,-3.43741114558699));
#455143=CARTESIAN_POINT('',(-4.21523428266519E-16,0.,-3.442));
#455144=CARTESIAN_POINT('Ctrl Pts',(0.00190492198109293,11.4223204546569,
-3.43753765796313));
#455145=CARTESIAN_POINT('Ctrl Pts',(0.447788094031521,11.4017650016966,
-3.43979577453365));
#455146=CARTESIAN_POINT('Ctrl Pts',(0.892886862129609,11.3812095487363,
-3.359223800869));
#455147=CARTESIAN_POINT('Ctrl Pts',(1.30262881999811,11.3606540957761,-3.19201212953924));
#455148=CARTESIAN_POINT('Ctrl Pts',(2.35423365298245,11.3078984204977,-2.76286251885132));
#455149=CARTESIAN_POINT('Ctrl Pts',(3.17294499666008,11.2551427452194,-1.76302167864693));
#455150=CARTESIAN_POINT('Ctrl Pts',(3.38623968972603,11.2023870699411,-0.647428792793382));
#455151=CARTESIAN_POINT('Ctrl Pts',(3.59953438279198,11.1496313946627,0.468164093060168));
#455152=CARTESIAN_POINT('Ctrl Pts',(3.20741242524624,11.0968757193844,1.69950902456289));
#455153=CARTESIAN_POINT('Ctrl Pts',(2.38829385790398,11.0441200441061,2.48632977012805));
#455154=CARTESIAN_POINT('Ctrl Pts',(1.56917529056172,10.9913643688278,3.27315051569321));
#455155=CARTESIAN_POINT('Ctrl Pts',(0.323060113422929,10.9386086935495,
3.61544707532083));
#455156=CARTESIAN_POINT('Ctrl Pts',(-0.783054809091477,10.8858530182711,
3.35747054250294));
#455157=CARTESIAN_POINT('Ctrl Pts',(-1.88916973160589,10.8330973429928,
3.09949400968504));
#455158=CARTESIAN_POINT('Ctrl Pts',(-2.85528439949591,10.7803416677145,
2.24124438442165));
#455159=CARTESIAN_POINT('Ctrl Pts',(-3.24180542797521,10.7275859924362,
1.17323520496348));
#455160=CARTESIAN_POINT('Ctrl Pts',(-3.62832645645451,10.6748303171578,
0.105226025505309));
#455161=CARTESIAN_POINT('Ctrl Pts',(-3.43525384552309,10.6220746418795,
-1.17254270814764));
#455162=CARTESIAN_POINT('Ctrl Pts',(-2.75043787476155,10.5693189666012,
-2.07867139598895));
#455163=CARTESIAN_POINT('Ctrl Pts',(-2.11438037556645,10.5203194626198,
-2.92028428433378));
#455164=CARTESIAN_POINT('Ctrl Pts',(-1.05411033988768,10.4713199586383,
-3.44129423348055));
#455165=CARTESIAN_POINT('Ctrl Pts',(0.00142507496518784,10.4223204546569,
-3.44683866470506));
#455166=CARTESIAN_POINT('Ctrl Pts',(0.00154693548059185,10.2776795453431,
-3.44670349103507));
#455167=CARTESIAN_POINT('Ctrl Pts',(-1.04641091131577,10.3263222110735,
-3.44080526105365));
#455168=CARTESIAN_POINT('Ctrl Pts',(-2.09936355514549,10.3749648768039,
-2.92834249274513));
#455169=CARTESIAN_POINT('Ctrl Pts',(-2.73639437423741,10.4236075425344,
-2.09712454699236));
#455170=CARTESIAN_POINT('Ctrl Pts',(-3.42728971333225,10.4763632178127,
-1.19562247318185));
#455171=CARTESIAN_POINT('Ctrl Pts',(-3.62895249796314,10.529118893091,0.0808188330383952));
#455172=CARTESIAN_POINT('Ctrl Pts',(-3.24962381232915,10.5818745683694,
1.15140376969445));
#455173=CARTESIAN_POINT('Ctrl Pts',(-2.87029512669516,10.6346302436477,
2.2219887063505));
#455174=CARTESIAN_POINT('Ctrl Pts',(-1.90997497079629,10.687385918926,3.08671727344235));
#455175=CARTESIAN_POINT('Ctrl Pts',(-0.805620163128287,10.7401415942043,
3.35212793737453));
#455176=CARTESIAN_POINT('Ctrl Pts',(0.298734644539725,10.7928972694826,
3.61753860130671));
#455177=CARTESIAN_POINT('Ctrl Pts',(1.54712410397688,10.845652944761,3.28363136207922));
#455178=CARTESIAN_POINT('Ctrl Pts',(2.37151652795347,10.8984086200393,2.50233788892262));
#455179=CARTESIAN_POINT('Ctrl Pts',(3.19590895193005,10.9511642953176,1.72104441576602));
#455180=CARTESIAN_POINT('Ctrl Pts',(3.59630434044607,11.0039199705959,0.49236470868034));
#455181=CARTESIAN_POINT('Ctrl Pts',(3.39051814454231,11.0566756458742,-0.62463770922453));
#455182=CARTESIAN_POINT('Ctrl Pts',(3.18473194863855,11.1094313211526,-1.7416401271294));
#455183=CARTESIAN_POINT('Ctrl Pts',(2.37276416831501,11.1621869964309,-2.74696525585346));
#455184=CARTESIAN_POINT('Ctrl Pts',(1.32406956584938,11.2149426717092,-3.18317849638681));
#455185=CARTESIAN_POINT('Ctrl Pts',(0.908368187698639,11.2358549629205,
-3.35609294147976));
#455186=CARTESIAN_POINT('Ctrl Pts',(0.455469431275188,11.2567672541318,
-3.43958165106471));
#455187=CARTESIAN_POINT('Ctrl Pts',(0.00180381072558041,11.2776795453431,
-3.43741114558699));
#455188=CARTESIAN_POINT('Origin',(0.,0.,0.));
#455189=CARTESIAN_POINT('',(-0.00294480074326642,12.4223204546569,-3.44006114644949));
#455190=CARTESIAN_POINT('',(-0.00298197493165331,12.2776795453431,-3.44027416367858));
#455191=CARTESIAN_POINT('',(-4.21523428266519E-16,0.,-3.442));
#455192=CARTESIAN_POINT('Ctrl Pts',(-0.00294480074326642,12.4223204546569,
-3.44006114644949));
#455193=CARTESIAN_POINT('Ctrl Pts',(0.805845936783274,12.3849657200332,
-3.43339405105818));
#455194=CARTESIAN_POINT('Ctrl Pts',(1.61886853933875,12.3476109854095,-3.14830562263054));
#455195=CARTESIAN_POINT('Ctrl Pts',(2.23183508531966,12.3102562507859,-2.62767871509275));
#455196=CARTESIAN_POINT('Ctrl Pts',(3.09752090485561,12.2575005755075,-1.89240313752745));
#455197=CARTESIAN_POINT('Ctrl Pts',(3.56418295590633,12.2047449002292,-0.687331977828459));
#455198=CARTESIAN_POINT('Ctrl Pts',(3.41948459040631,12.1519892249509,0.439213403454665));
#455199=CARTESIAN_POINT('Ctrl Pts',(3.2747862249063,12.0992335496726,1.56575878473779));
#455200=CARTESIAN_POINT('Ctrl Pts',(2.51872744285554,12.0464778743942,2.61377838760505));
#455201=CARTESIAN_POINT('Ctrl Pts',(1.49532376292829,11.9937221991159,3.10641113213925));
#455202=CARTESIAN_POINT('Ctrl Pts',(0.471920083001049,11.9409665238376,
3.59904387667346));
#455203=CARTESIAN_POINT('Ctrl Pts',(-0.81882849480268,11.8882108485593,
3.53628976287462));
#455204=CARTESIAN_POINT('Ctrl Pts',(-1.78961639050565,11.835455173281,2.94670264069157));
#455205=CARTESIAN_POINT('Ctrl Pts',(-2.76040428620862,11.7826994980026,
2.35711551850853));
#455206=CARTESIAN_POINT('Ctrl Pts',(-3.41123149981084,11.7299438227243,
1.24069538794127));
#455207=CARTESIAN_POINT('Ctrl Pts',(-3.44596409730449,11.677188147446,0.105426362666967));
#455208=CARTESIAN_POINT('Ctrl Pts',(-3.48069669479813,11.6244324721677,
-1.02984266260733));
#455209=CARTESIAN_POINT('Ctrl Pts',(-2.89933467618322,11.5716767968893,
-2.18396058258869));
#455210=CARTESIAN_POINT('Ctrl Pts',(-1.96640450573024,11.518921121611,-2.83179035199364));
#455211=CARTESIAN_POINT('Ctrl Pts',(-1.39697650130591,11.486720899293,-3.22720302539858));
#455212=CARTESIAN_POINT('Ctrl Pts',(-0.696573350214575,11.4545206769749,
-3.43400030679256));
#455213=CARTESIAN_POINT('Ctrl Pts',(0.00190492198109293,11.4223204546569,
-3.43753765796313));
#455214=CARTESIAN_POINT('Ctrl Pts',(0.00180381072558041,11.2776795453431,
-3.43741114558699));
#455215=CARTESIAN_POINT('Ctrl Pts',(-0.688997997991005,11.3095229294101,
-3.43410609216896));
#455216=CARTESIAN_POINT('Ctrl Pts',(-1.38157789620168,11.3413663134772,
-3.23218730108958));
#455217=CARTESIAN_POINT('Ctrl Pts',(-1.94731304484871,11.3732096975442,
-2.8449529803043));
#455218=CARTESIAN_POINT('Ctrl Pts',(-2.88457962847346,11.4259653728225,
-2.20341287134578));
#455219=CARTESIAN_POINT('Ctrl Pts',(-3.47369137111525,11.4787210481008,
-1.05323130108607));
#455220=CARTESIAN_POINT('Ctrl Pts',(-3.44659559399869,11.5314767233792,
0.0822457700539528));
#455221=CARTESIAN_POINT('Ctrl Pts',(-3.41949981688212,11.5842323986575,
1.21772284119398));
#455222=CARTESIAN_POINT('Ctrl Pts',(-2.7761965200072,11.6369880739358,2.33849541321433));
#455223=CARTESIAN_POINT('Ctrl Pts',(-1.80939616804833,11.6897437492141,
2.93459896103683));
#455224=CARTESIAN_POINT('Ctrl Pts',(-0.842595816089467,11.7424994244925,
3.53070250885933));
#455225=CARTESIAN_POINT('Ctrl Pts',(0.447701590953337,11.7952550997708,
3.60213703248398));
#455226=CARTESIAN_POINT('Ctrl Pts',(1.47439576108161,11.8480107750491,3.1163989947945));
#455227=CARTESIAN_POINT('Ctrl Pts',(2.50108993120989,11.9007664503274,2.63066095710503));
#455228=CARTESIAN_POINT('Ctrl Pts',(3.26418086442365,11.9535221256058,1.58775035810145));
#455229=CARTESIAN_POINT('Ctrl Pts',(3.41645333163715,12.0062778008841,0.462203621635271));
#455230=CARTESIAN_POINT('Ctrl Pts',(3.56872579885066,12.0590334761624,-0.663343114830906));
#455231=CARTESIAN_POINT('Ctrl Pts',(3.11017980006393,12.1117891514407,-1.87152598875967));
#455232=CARTESIAN_POINT('Ctrl Pts',(2.24945908542769,12.164544826719,-2.61260777348285));
#455233=CARTESIAN_POINT('Ctrl Pts',(1.63418628712663,12.2022563995937,-3.14235854594947));
#455234=CARTESIAN_POINT('Ctrl Pts',(0.813406931721569,12.2399679724684,
-3.43342614695064));
#455235=CARTESIAN_POINT('Ctrl Pts',(-0.00298197493165331,12.2776795453431,
-3.44027416367858));
#455236=CARTESIAN_POINT('Origin',(0.,0.,0.));
#455237=CARTESIAN_POINT('',(0.000551455541893276,13.4223204546569,-3.44746546819473));
#455238=CARTESIAN_POINT('',(0.000689626542513858,13.2776795453431,-3.44740402518832));
#455239=CARTESIAN_POINT('',(-4.21523428266519E-16,0.,-3.442));
#455240=CARTESIAN_POINT('Ctrl Pts',(0.000551455541893276,13.4223204546569,
-3.44746546819473));
#455241=CARTESIAN_POINT('Ctrl Pts',(0.0306595665508508,13.4209221136481,
-3.44753286857709));
#455242=CARTESIAN_POINT('Ctrl Pts',(0.0607660228121984,13.4195237726394,
-3.44717233639977));
#455243=CARTESIAN_POINT('Ctrl Pts',(0.0908610660097724,13.4181254316307,
-3.44637890430166));
#455244=CARTESIAN_POINT('Ctrl Pts',(1.22626674780566,13.3653697563523,-3.41644482823507));
#455245=CARTESIAN_POINT('Ctrl Pts',(2.34542762737645,13.312614081074,-2.77034197086878));
#455246=CARTESIAN_POINT('Ctrl Pts',(2.93911251532146,13.2598584057957,-1.80205463313301));
#455247=CARTESIAN_POINT('Ctrl Pts',(3.53279740326646,13.2071027305174,-0.833767295397236));
#455248=CARTESIAN_POINT('Ctrl Pts',(3.60100629958569,13.154347055239,0.456704522708029));
#455249=CARTESIAN_POINT('Ctrl Pts',(3.11270336662071,13.1015913799607,1.48218117207498));
#455250=CARTESIAN_POINT('Ctrl Pts',(2.62440043365574,13.0488357046824,2.50765782144194));
#455251=CARTESIAN_POINT('Ctrl Pts',(1.57958567140657,12.9960800294041,3.26813930207059));
#455252=CARTESIAN_POINT('Ctrl Pts',(0.453661919259777,12.9433243541257,
3.41759771506665));
#455253=CARTESIAN_POINT('Ctrl Pts',(-0.672261832887001,12.8905686788474,
3.5670561280627));
#455254=CARTESIAN_POINT('Ctrl Pts',(-1.8792945749314,12.8378130035691,3.10549147342618));
#455255=CARTESIAN_POINT('Ctrl Pts',(-2.61822240311915,12.7850573282908,
2.24292102527514));
#455256=CARTESIAN_POINT('Ctrl Pts',(-3.3571502313069,12.7323016530125,1.38035057712408));
#455257=CARTESIAN_POINT('Ctrl Pts',(-3.62797314563799,12.6795459777341,
0.116774335458481));
#455258=CARTESIAN_POINT('Ctrl Pts',(-3.30746357785179,12.6267903024558,
-0.972865848260009));
#455259=CARTESIAN_POINT('Ctrl Pts',(-2.9869540100656,12.5740346271775,-2.0625060319785));
#455260=CARTESIAN_POINT('Ctrl Pts',(-2.07511196016212,12.5212789518992,
-2.97821015774988));
#455261=CARTESIAN_POINT('Ctrl Pts',(-0.986836141199789,12.4685232766208,
-3.30332222291977));
#455262=CARTESIAN_POINT('Ctrl Pts',(-0.669136268810636,12.4531223359662,
-3.39823204248659));
#455263=CARTESIAN_POINT('Ctrl Pts',(-0.336400205423888,12.4377213953115,
-3.44280991555452));
#455264=CARTESIAN_POINT('Ctrl Pts',(-0.00294480074326642,12.4223204546569,
-3.44006114644949));
#455265=CARTESIAN_POINT('Ctrl Pts',(-0.00298197493165331,12.2776795453431,
-3.44027416367858));
#455266=CARTESIAN_POINT('Ctrl Pts',(-0.328660205158152,12.2927236477467,
-3.44300601114777));
#455267=CARTESIAN_POINT('Ctrl Pts',(-0.653639733070962,12.3077677501504,
-3.40050674618356));
#455268=CARTESIAN_POINT('Ctrl Pts',(-0.964595131274779,12.322811852554,
-3.3098854644577));
#455269=CARTESIAN_POINT('Ctrl Pts',(-2.05503320285527,12.3755675278323,
-2.9921006751918));
#455270=CARTESIAN_POINT('Ctrl Pts',(-2.97301391553049,12.4283232031107,
-2.08255040114239));
#455271=CARTESIAN_POINT('Ctrl Pts',(-3.30084539334331,12.481078878389,-0.995090570900892));
#455272=CARTESIAN_POINT('Ctrl Pts',(-3.62867687115614,12.5338345536673,
0.0923692593406071));
#455273=CARTESIAN_POINT('Ctrl Pts',(-3.36635911410655,12.5865902289456,
1.35773864577421));
#455274=CARTESIAN_POINT('Ctrl Pts',(-2.63324974540749,12.6393459042239,
2.22525983502552));
#455275=CARTESIAN_POINT('Ctrl Pts',(-1.90014037670843,12.6921015795023,
3.09278102427684));
#455276=CARTESIAN_POINT('Ctrl Pts',(-0.69623939635987,12.7448572547806,
3.56245401634588));
#455277=CARTESIAN_POINT('Ctrl Pts',(0.430664280185392,12.7976129300589,
3.42057214995318));
#455278=CARTESIAN_POINT('Ctrl Pts',(1.55756795673064,12.8503686053373,3.27869028356049));
#455279=CARTESIAN_POINT('Ctrl Pts',(2.60747432947258,12.9031242806156,2.52525355870611));
#455280=CARTESIAN_POINT('Ctrl Pts',(3.10266381641936,12.9558799558939,1.50308442778917));
#455281=CARTESIAN_POINT('Ctrl Pts',(3.59785330336615,13.0086356311722,0.480915296872219));
#455282=CARTESIAN_POINT('Ctrl Pts',(3.53832590451775,13.0613913064505,-0.809986240107284));
#455283=CARTESIAN_POINT('Ctrl Pts',(2.95116727689351,13.1141469817289,-1.78224500528432));
#455284=CARTESIAN_POINT('Ctrl Pts',(2.36400864926926,13.1669026570072,-2.75450377046135));
#455285=CARTESIAN_POINT('Ctrl Pts',(1.24921879286915,13.2196583322855,-3.40811976383592));
#455286=CARTESIAN_POINT('Ctrl Pts',(0.114040028051502,13.2724140075638,
-3.44569012365563));
#455287=CARTESIAN_POINT('Ctrl Pts',(0.0762726748025813,13.2741691868236,
-3.44694008806209));
#455288=CARTESIAN_POINT('Ctrl Pts',(0.038482753268587,13.2759243660833,
-3.44750815752882));
#455289=CARTESIAN_POINT('Ctrl Pts',(0.000689626542513858,13.2776795453431,
-3.44740402518832));
#455290=CARTESIAN_POINT('Origin',(0.,0.,0.));
#455291=CARTESIAN_POINT('',(0.00248787001207174,14.4223204546569,-3.43854544754782));
#455292=CARTESIAN_POINT('',(0.00241009727763581,14.2776795453431,-3.43837553245923));
#455293=CARTESIAN_POINT('',(-4.21523428266519E-16,0.,-3.442));
#455294=CARTESIAN_POINT('Ctrl Pts',(0.00248787001207174,14.4223204546569,
-3.43854544754782));
#455295=CARTESIAN_POINT('Ctrl Pts',(0.396934926497801,14.4041228319848,
-3.44120536324132));
#455296=CARTESIAN_POINT('Ctrl Pts',(0.790562293081628,14.3859252093126,
-3.37850410109726));
#455297=CARTESIAN_POINT('Ctrl Pts',(1.15952320178319,14.3677275866405,-3.24673520366357));
#455298=CARTESIAN_POINT('Ctrl Pts',(2.22915643028483,14.3149719113622,-2.8647316150609));
#455299=CARTESIAN_POINT('Ctrl Pts',(3.09148175965367,14.2622162360838,-1.90225285493972));
#455300=CARTESIAN_POINT('Ctrl Pts',(3.35413100037242,14.2094605608055,-0.797238122286408));
#455301=CARTESIAN_POINT('Ctrl Pts',(3.61678024109116,14.1567048855272,0.307776610366904));
#455302=CARTESIAN_POINT('Ctrl Pts',(3.27975339315982,14.1039492102489,1.55532731555235));
#455303=CARTESIAN_POINT('Ctrl Pts',(2.49640166552181,14.0511935349705,2.37776404794338));
#455304=CARTESIAN_POINT('Ctrl Pts',(1.71304993788381,13.9984378596922,3.20020078033441));
#455305=CARTESIAN_POINT('Ctrl Pts',(0.483373330539141,13.9456821844139,
3.59752353993101));
#455306=CARTESIAN_POINT('Ctrl Pts',(-0.633111074588675,13.8929265091356,
3.38894580815677));
#455307=CARTESIAN_POINT('Ctrl Pts',(-1.74959547971649,13.8401708338572,
3.18036807638253));
#455308=CARTESIAN_POINT('Ctrl Pts',(-2.75288768262745,13.7874151585789,
2.36588985323744));
#455309=CARTESIAN_POINT('Ctrl Pts',(-3.18647806713122,13.7346594833006,
1.31610820833249));
#455310=CARTESIAN_POINT('Ctrl Pts',(-3.62006845163498,13.6819038080223,
0.266326563427543));
#455311=CARTESIAN_POINT('Ctrl Pts',(-3.48395701773154,13.6291481327439,
-1.01875850323727));
#455312=CARTESIAN_POINT('Ctrl Pts',(-2.84007605876933,13.5763924574656,
-1.95441838918622));
#455313=CARTESIAN_POINT('Ctrl Pts',(-2.21326179727459,13.525035123196,-2.86527769051828));
#455314=CARTESIAN_POINT('Ctrl Pts',(-1.10523912890168,13.4736777889265,
-3.44499003198518));
#455315=CARTESIAN_POINT('Ctrl Pts',(0.000551455541893276,13.4223204546569,
-3.44746546819473));
#455316=CARTESIAN_POINT('Ctrl Pts',(0.000689626542513858,13.2776795453431,
-3.44740402518832));
#455317=CARTESIAN_POINT('Ctrl Pts',(-1.0974706886562,13.3286800413617,-3.44437823680371));
#455318=CARTESIAN_POINT('Ctrl Pts',(-2.1983372039437,13.3796805373802,-2.87380063074141));
#455319=CARTESIAN_POINT('Ctrl Pts',(-2.82686629247264,13.4306810333988,
-1.9734772654318));
#455320=CARTESIAN_POINT('Ctrl Pts',(-3.47702617494399,13.4834367086771,
-1.04216932112342));
#455321=CARTESIAN_POINT('Ctrl Pts',(-3.62177826665152,13.5361923839554,
0.241971293758206));
#455322=CARTESIAN_POINT('Ctrl Pts',(-3.19525868498632,13.5889480592338,
1.29464570125774));
#455323=CARTESIAN_POINT('Ctrl Pts',(-2.76873910332111,13.6417037345121,
2.34732010875727));
#455324=CARTESIAN_POINT('Ctrl Pts',(-1.77094784828316,13.6944594097904,
3.1685283088747));
#455325=CARTESIAN_POINT('Ctrl Pts',(-0.655891521124064,13.7472150850688,
3.38461103748138));
#455326=CARTESIAN_POINT('Ctrl Pts',(0.459164806035046,13.7999707603471,
3.60069376608806));
#455327=CARTESIAN_POINT('Ctrl Pts',(1.69148620531532,13.8527264356254,3.21165102318395));
#455328=CARTESIAN_POINT('Ctrl Pts',(2.4803521456137,13.9054821109037,2.39450177922372));
#455329=CARTESIAN_POINT('Ctrl Pts',(3.26921808591208,13.958237786182,1.57735253526349));
#455330=CARTESIAN_POINT('Ctrl Pts',(3.6146285672286,14.0109934614604,0.332096790247161));
#455331=CARTESIAN_POINT('Ctrl Pts',(3.35941780359704,14.0637491367387,-0.774659658454042));
#455332=CARTESIAN_POINT('Ctrl Pts',(3.10420703996547,14.116504812017,-1.88141610715523));
#455333=CARTESIAN_POINT('Ctrl Pts',(2.24837503138585,14.1692604872953,-2.84967325954128));
#455334=CARTESIAN_POINT('Ctrl Pts',(1.18133528971154,14.2220161625737,-3.2388628457514));
#455335=CARTESIAN_POINT('Ctrl Pts',(0.806051548466779,14.2405706234968,
-3.37574296207889));
#455336=CARTESIAN_POINT('Ctrl Pts',(0.404642095862786,14.2591250844199,
-3.44099429914845));
#455337=CARTESIAN_POINT('Ctrl Pts',(0.00241009727763581,14.2776795453431,
-3.43837553245923));
#455338=CARTESIAN_POINT('Origin',(0.,0.,0.));
#455339=CARTESIAN_POINT('',(-0.00257283171653078,15.4223204546569,-3.43875668620077));
#455340=CARTESIAN_POINT('',(-0.00264566132197309,15.2776795453431,-3.43894503739979));
#455341=CARTESIAN_POINT('',(-4.21523428266519E-16,0.,-3.442));
#455342=CARTESIAN_POINT('Ctrl Pts',(-0.00257283171653078,15.4223204546569,
-3.43875668620077));
#455343=CARTESIAN_POINT('Ctrl Pts',(0.755888892797501,15.3873235503214,
-3.43343588809486));
#455344=CARTESIAN_POINT('Ctrl Pts',(1.5175038776905,15.3523266459858,-3.18601278121568));
#455345=CARTESIAN_POINT('Ctrl Pts',(2.11288261599305,15.3173297416503,-2.72424597002973));
#455346=CARTESIAN_POINT('Ctrl Pts',(3.01037935125762,15.264574066372,-2.02816097600645));
#455347=CARTESIAN_POINT('Ctrl Pts',(3.53012577026604,15.2118183910936,-0.845007705659107));
#455348=CARTESIAN_POINT('Ctrl Pts',(3.43562315009899,15.1590627158153,0.286855454432574));
#455349=CARTESIAN_POINT('Ctrl Pts',(3.34112052993194,15.106307040537,1.41871861452425));
#455350=CARTESIAN_POINT('Ctrl Pts',(2.63236887058942,15.0535513652587,2.49929166436027));
#455351=CARTESIAN_POINT('Ctrl Pts',(1.63186259450475,15.0007956899804,3.03690648184037));
#455352=CARTESIAN_POINT('Ctrl Pts',(0.631356318420086,14.948040014702,3.57452129932047));
#455353=CARTESIAN_POINT('Ctrl Pts',(-0.66090457440673,14.8952843394237,
3.56917788444466));
#455354=CARTESIAN_POINT('Ctrl Pts',(-1.65692856184199,14.8425286641454,
3.02330487528562));
#455355=CARTESIAN_POINT('Ctrl Pts',(-2.65295254927725,14.7897729888671,
2.47743186612658));
#455356=CARTESIAN_POINT('Ctrl Pts',(-3.35273963132095,14.7370173135887,
1.39102926268431));
#455357=CARTESIAN_POINT('Ctrl Pts',(-3.43787743377992,14.6842616383104,
0.258424246683737));
#455358=CARTESIAN_POINT('Ctrl Pts',(-3.52301523623888,14.6315059630321,
-0.87418076931683));
#455359=CARTESIAN_POINT('Ctrl Pts',(-2.99350375911311,14.5787502877538,
-2.0529881978757));
#455360=CARTESIAN_POINT('Ctrl Pts',(-2.090277456733,14.5259946124754,-2.74162770361305));
#455361=CARTESIAN_POINT('Ctrl Pts',(-1.49861140548322,14.4914365598693,
-3.19272685342806));
#455362=CARTESIAN_POINT('Ctrl Pts',(-0.746583718842133,14.4568785072631,
-3.43349415551258));
#455363=CARTESIAN_POINT('Ctrl Pts',(0.00248787001207174,14.4223204546569,
-3.43854544754782));
#455364=CARTESIAN_POINT('Ctrl Pts',(0.00241009727763581,14.2776795453431,
-3.43837553245923));
#455365=CARTESIAN_POINT('Ctrl Pts',(-0.739019301350593,14.3118807596983,
-3.43354839136065));
#455366=CARTESIAN_POINT('Ctrl Pts',(-1.48324347308736,14.3460819740534,
-3.19811828677568));
#455367=CARTESIAN_POINT('Ctrl Pts',(-2.07178973503114,14.3802831884086,
-2.7556256485914));
#455368=CARTESIAN_POINT('Ctrl Pts',(-2.97962754333046,14.4330388636869,
-2.0730768451871));
#455369=CARTESIAN_POINT('Ctrl Pts',(-3.51705568516008,14.4857945389653,
-0.897857218344334));
#455370=CARTESIAN_POINT('Ctrl Pts',(-3.43953805554209,14.5385502142436,
0.235294778045084));
#455371=CARTESIAN_POINT('Ctrl Pts',(-3.36202042592409,14.5913058895219,
1.3684467744345));
#455372=CARTESIAN_POINT('Ctrl Pts',(-2.66955702485847,14.6440615648002,
2.45953114037057));
#455373=CARTESIAN_POINT('Ctrl Pts',(-1.67722685885009,14.6968172400786,
3.01209161175412));
#455374=CARTESIAN_POINT('Ctrl Pts',(-0.684896692841708,14.7495729153569,
3.56465208313766));
#455375=CARTESIAN_POINT('Ctrl Pts',(0.607300238109442,14.8023285906352,
3.57868865996868));
#455376=CARTESIAN_POINT('Ctrl Pts',(1.6113995754516,14.8550842659135,3.04781495530594));
#455377=CARTESIAN_POINT('Ctrl Pts',(2.61549891279374,14.9078399411919,2.5169412506432));
#455378=CARTESIAN_POINT('Ctrl Pts',(3.3315006565269,14.9605956164702,1.44115726448671));
#455379=CARTESIAN_POINT('Ctrl Pts',(3.43361524521218,15.0133512917485,0.309956387754804));
#455380=CARTESIAN_POINT('Ctrl Pts',(3.53572983389747,15.0661069670268,-0.821244488977105));
#455381=CARTESIAN_POINT('Ctrl Pts',(3.02395726753487,15.1188626423052,-2.00786225628442));
#455382=CARTESIAN_POINT('Ctrl Pts',(2.13116088774389,15.1716183175835,-2.70997051031363));
#455383=CARTESIAN_POINT('Ctrl Pts',(1.53286140191971,15.20697206017,-3.18048205906893));
#455384=CARTESIAN_POINT('Ctrl Pts',(0.763448312546386,15.2423258027566,
-3.43340571476085));
#455385=CARTESIAN_POINT('Ctrl Pts',(-0.00264566132197309,15.2776795453431,
-3.43894503739979));
#455386=CARTESIAN_POINT('Origin',(0.,0.,0.));
#455387=CARTESIAN_POINT('',(-0.000142136989979558,16.4223204546569,-3.44723320560186));
#455388=CARTESIAN_POINT('',(-0.000213030569266609,16.2776795453431,-3.44751024702897));
#455389=CARTESIAN_POINT('',(-4.21523428266519E-16,0.,-3.442));
#455390=CARTESIAN_POINT('Ctrl Pts',(-0.000142136989979558,16.4223204546569,
-3.44723320560186));
#455391=CARTESIAN_POINT('Ctrl Pts',(1.11523026578114,16.370524268658,-3.44525091864187));
#455392=CARTESIAN_POINT('Ctrl Pts',(2.23158337703984,16.318728082659,-2.85471407152575));
#455393=CARTESIAN_POINT('Ctrl Pts',(2.85602730912618,16.2669318966601,-1.93100385516442));
#455394=CARTESIAN_POINT('Ctrl Pts',(3.49203864230329,16.2141762213818,-0.990182532400653));
#455395=CARTESIAN_POINT('Ctrl Pts',(3.61774742836716,16.1614205461035,0.29627011044174));
#455396=CARTESIAN_POINT('Ctrl Pts',(3.17554384765381,16.1086648708251,1.34249779760182));
#455397=CARTESIAN_POINT('Ctrl Pts',(2.73334026694047,16.0559091955468,2.38872548476189));
#455398=CARTESIAN_POINT('Ctrl Pts',(1.72322431944992,16.0031535202685,3.19472821623966));
#455399=CARTESIAN_POINT('Ctrl Pts',(0.605023750021618,15.9503978449902,
3.39402755401468));
#455400=CARTESIAN_POINT('Ctrl Pts',(-0.513176819406664,15.8976421697119,
3.59332689178971));
#455401=CARTESIAN_POINT('Ctrl Pts',(-1.73946201077269,15.8448864944335,
3.18592283586202));
#455402=CARTESIAN_POINT('Ctrl Pts',(-2.51596861503884,15.7921308191552,
2.35705280052856));
#455403=CARTESIAN_POINT('Ctrl Pts',(-3.29247521930499,15.7393751438769,
1.5281827651951));
#455404=CARTESIAN_POINT('Ctrl Pts',(-3.61920323647126,15.6866194685986,
0.277846750455868));
#455405=CARTESIAN_POINT('Ctrl Pts',(-3.34743007316696,15.6338637933202,
-0.824967112775094));
#455406=CARTESIAN_POINT('Ctrl Pts',(-3.07565690986267,15.5811081180419,
-1.92778097600606));
#455407=CARTESIAN_POINT('Ctrl Pts',(-2.2053825660878,15.5283524427636,-2.88307268772875));
#455408=CARTESIAN_POINT('Ctrl Pts',(-1.13262186844002,15.4755967674853,
-3.25621018474049));
#455409=CARTESIAN_POINT('Ctrl Pts',(-0.771505999759574,15.4578379965425,
-3.38181682904251));
#455410=CARTESIAN_POINT('Ctrl Pts',(-0.387445388025546,15.4400792255997,
-3.44145666314416));
#455411=CARTESIAN_POINT('Ctrl Pts',(-0.00257283171653078,15.4223204546569,
-3.43875668620077));
#455412=CARTESIAN_POINT('Ctrl Pts',(-0.00264566132197309,15.2776795453431,
-3.43894503739979));
#455413=CARTESIAN_POINT('Ctrl Pts',(-0.379734896958102,15.2950814780349,
-3.44167162057511));
#455414=CARTESIAN_POINT('Ctrl Pts',(-0.756019965044454,15.3124834107267,
-3.38446101486161));
#455415=CARTESIAN_POINT('Ctrl Pts',(-1.11069842846604,15.3298853434184,
-3.26375976668423));
#455416=CARTESIAN_POINT('Ctrl Pts',(-2.18594117166558,15.3826410186968,
-2.89784202827451));
#455417=CARTESIAN_POINT('Ctrl Pts',(-3.06260646484528,15.4353966939751,
-1.94840781070399));
#455418=CARTESIAN_POINT('Ctrl Pts',(-3.34179814439852,15.4881523692534,
-0.847454950509992));
#455419=CARTESIAN_POINT('Ctrl Pts',(-3.62098982395176,15.5409080445317,
0.253497909683986));
#455420=CARTESIAN_POINT('Ctrl Pts',(-3.30270788987855,15.5936637198101,
1.50596941250144));
#455421=CARTESIAN_POINT('Ctrl Pts',(-2.53178063602364,15.6464193950884,
2.34005942226194));
#455422=CARTESIAN_POINT('Ctrl Pts',(-1.76085338216871,15.6991750703667,
3.17414943202246));
#455423=CARTESIAN_POINT('Ctrl Pts',(-0.537280808532051,15.751930745645,
3.58985794872603));
#455424=CARTESIAN_POINT('Ctrl Pts',(0.582209535696286,15.8046864209234,
3.39805408507685));
#455425=CARTESIAN_POINT('Ctrl Pts',(1.70169987992463,15.8574420962017,3.20625022142767));
#455426=CARTESIAN_POINT('Ctrl Pts',(2.71710799474464,15.91019777148,2.40693397742575));
#455427=CARTESIAN_POINT('Ctrl Pts',(3.16638797553546,15.9629534467583,1.36376248720178));
#455428=CARTESIAN_POINT('Ctrl Pts',(3.61566795632629,16.0157091220366,0.320590996977814));
#455429=CARTESIAN_POINT('Ctrl Pts',(3.49881980308792,16.068464797315,-0.966435739468192));
#455430=CARTESIAN_POINT('Ctrl Pts',(2.8690558925296,16.1212204725933,-1.9116266225805));
#455431=CARTESIAN_POINT('Ctrl Pts',(2.24648604908041,16.1733734968432,-2.84602017905969));
#455432=CARTESIAN_POINT('Ctrl Pts',(1.12265203508462,16.2255265210932,-3.44634315369573));
#455433=CARTESIAN_POINT('Ctrl Pts',(-0.000213030569266609,16.2776795453431,
-3.44751024702897));
#455434=CARTESIAN_POINT('Origin',(0.,5.25141010809499,0.));
#455435=CARTESIAN_POINT('',(-0.000118598906288441,16.751410108095,-2.87636657945628));
#455436=CARTESIAN_POINT('',(-1.47936051206424E-13,16.9,-2.872));
#455437=CARTESIAN_POINT('',(-1.47936051206424E-13,5.25141010809499,-2.872));
#455438=CARTESIAN_POINT('',(-2.30844912129813,16.9,-1.70863883087617));
#455439=CARTESIAN_POINT('Ctrl Pts',(-0.00011859890628823,16.751410108095,
-2.87636657945628));
#455440=CARTESIAN_POINT('Ctrl Pts',(-0.0173585412542118,16.7523695973744,
-2.87639721901023));
#455441=CARTESIAN_POINT('Ctrl Pts',(-0.907290126313184,16.8018995613427,
-2.86927979781993));
#455442=CARTESIAN_POINT('Ctrl Pts',(-1.78950708297451,16.8514295253111,
-2.40949662694586));
#455443=CARTESIAN_POINT('Ctrl Pts',(-2.312781279227,16.9,-1.71040874167461));
#455444=CARTESIAN_POINT('Origin',(0.,16.9,0.));
#455445=CARTESIAN_POINT('Origin',(0.,5.25141010809499,0.));
#455446=CARTESIAN_POINT('',(-0.00214676719638619,15.751410108095,-2.86929378348885));
#455447=CARTESIAN_POINT('',(-0.00017775241010487,15.948589891905,-2.87659774243672));
#455448=CARTESIAN_POINT('',(-1.47936051206424E-13,5.25141010809499,-2.872));
#455449=CARTESIAN_POINT('Ctrl Pts',(-0.00214676719638623,15.751410108095,
-2.86929378348885));
#455450=CARTESIAN_POINT('Ctrl Pts',(-0.323283891461201,15.7691688790378,
-2.87154664048518));
#455451=CARTESIAN_POINT('Ctrl Pts',(-1.59572746551707,15.8396833252589,
-2.67395198656385));
#455452=CARTESIAN_POINT('Ctrl Pts',(-3.29247953528384,15.9629534467583,
-0.811443685944723));
#455453=CARTESIAN_POINT('Ctrl Pts',(-2.47461532961719,16.1212204725933,
2.31839219522703));
#455454=CARTESIAN_POINT('Ctrl Pts',(0.595016631106169,16.2794874984283,
3.33820432360382));
#455455=CARTESIAN_POINT('Ctrl Pts',(3.12353464492909,16.4377545242632,1.32062165817314));
#455456=CARTESIAN_POINT('Ctrl Pts',(2.81076863784611,16.5950620608188,-1.88009858582563));
#455457=CARTESIAN_POINT('Ctrl Pts',(0.930546578536684,16.6996139220961,
-2.87471256198127));
#455458=CARTESIAN_POINT('Ctrl Pts',(-0.00011859890628823,16.751410108095,
-2.87636657945628));
#455459=CARTESIAN_POINT('',(0.863261863496793,16.9,-2.73919020059434));
#455460=CARTESIAN_POINT('Origin',(0.,16.9,0.));
#455461=CARTESIAN_POINT('Ctrl Pts',(-0.000177752410104636,15.948589891905,
-2.87659774243672));
#455462=CARTESIAN_POINT('Ctrl Pts',(-0.0110042390567035,15.9491925429334,
-2.8766089953653));
#455463=CARTESIAN_POINT('Ctrl Pts',(-0.969564698895354,16.0025508692401,
-2.87169484567401));
#455464=CARTESIAN_POINT('Ctrl Pts',(-2.86409573659214,16.1086648708252,
-1.81589248079735));
#455465=CARTESIAN_POINT('Ctrl Pts',(-3.08280821480706,16.2669318966601,
1.4122865025187));
#455466=CARTESIAN_POINT('Ctrl Pts',(-0.497155858873794,16.4251989224951,
3.35338935516332));
#455467=CARTESIAN_POINT('Ctrl Pts',(2.54297493246889,16.58346594833,2.24645259117239));
#455468=CARTESIAN_POINT('Ctrl Pts',(3.26488853074936,16.741732974165,-0.912123640571359));
#455469=CARTESIAN_POINT('Ctrl Pts',(1.77123132985941,16.8472443247217,-2.45304161063505));
#455470=CARTESIAN_POINT('Ctrl Pts',(0.863261863496793,16.9,-2.73919020059434));
#455471=CARTESIAN_POINT('Origin',(0.,5.25141010809499,0.));
#455472=CARTESIAN_POINT('',(0.00207587526855749,14.751410108095,-2.8691175262514));
#455473=CARTESIAN_POINT('',(-0.00220753611772651,14.948589891905,-2.86945094346665));
#455474=CARTESIAN_POINT('',(-1.47936051206424E-13,5.25141010809499,-2.872));
#455475=CARTESIAN_POINT('Ctrl Pts',(0.00207587526855756,14.751410108095,
-2.8691175262514));
#455476=CARTESIAN_POINT('Ctrl Pts',(-0.622948413862524,14.7859681607012,
-2.8649027352214));
#455477=CARTESIAN_POINT('Ctrl Pts',(-2.20835504002284,14.8732818885857,
-2.3573229175255));
#455478=CARTESIAN_POINT('Ctrl Pts',(-3.38142263822873,15.0133512917485,
0.254180059658117));
#455479=CARTESIAN_POINT('Ctrl Pts',(-1.62971854209606,15.1716183175835,
2.97365851150546));
#455480=CARTESIAN_POINT('Ctrl Pts',(1.60506351850703,15.3298853434185,2.98703412526777));
#455481=CARTESIAN_POINT('Ctrl Pts',(3.37920770702971,15.4881523692534,0.282148187618979));
#455482=CARTESIAN_POINT('Ctrl Pts',(2.22416583374883,15.6286606241456,-2.34719473766286));
#455483=CARTESIAN_POINT('Ctrl Pts',(0.630712638034381,15.7164132037595,
-2.86485411696934));
#455484=CARTESIAN_POINT('Ctrl Pts',(-0.00214676719638623,15.751410108095,
-2.86929378348885));
#455485=CARTESIAN_POINT('Ctrl Pts',(-0.0022075361177263,14.948589891905,
-2.86945094346665));
#455486=CARTESIAN_POINT('Ctrl Pts',(-0.316850268467174,14.9659918245968,
-2.87172600066579));
#455487=CARTESIAN_POINT('Ctrl Pts',(-1.58265828892416,15.0361494325669,
-2.6792717958374));
#455488=CARTESIAN_POINT('Ctrl Pts',(-3.28692286143165,15.1590627158153,
-0.833542173003866));
#455489=CARTESIAN_POINT('Ctrl Pts',(-2.49020085562839,15.3173297416503,
2.30163925299127));
#455490=CARTESIAN_POINT('Ctrl Pts',(0.572640891743325,15.4755967674853,
3.34223907283957));
#455491=CARTESIAN_POINT('Ctrl Pts',(3.11440623668499,15.6338637933202,1.34139399488469));
#455492=CARTESIAN_POINT('Ctrl Pts',(2.82302618968387,15.7915281681268,-1.8680183968737));
#455493=CARTESIAN_POINT('Ctrl Pts',(0.936739292493483,15.8964368676551,
-2.87562392138709));
#455494=CARTESIAN_POINT('Ctrl Pts',(-0.000177752410104636,15.948589891905,
-2.87659774243672));
#455495=CARTESIAN_POINT('Origin',(0.,5.25141010809499,0.));
#455496=CARTESIAN_POINT('',(0.000460133735044288,13.751410108095,-2.87656037903988));
#455497=CARTESIAN_POINT('',(0.00201098180729872,13.948589891905,-2.86897574933844));
#455498=CARTESIAN_POINT('',(-1.47936051206424E-13,5.25141010809499,-2.872));
#455499=CARTESIAN_POINT('Ctrl Pts',(0.000460133735044324,13.751410108095,
-2.87656037903988));
#455500=CARTESIAN_POINT('Ctrl Pts',(-0.922209987857596,13.8027674423646,
-2.87449487851869));
#455501=CARTESIAN_POINT('Ctrl Pts',(-2.79644800244617,13.9068804519124,
-1.89390220752309));
#455502=CARTESIAN_POINT('Ctrl Pts',(-3.13415125835744,14.0637491367387,
1.29449570064652));
#455503=CARTESIAN_POINT('Ctrl Pts',(-0.622714413418182,14.2220161625736,
3.33329418136064));
#455504=CARTESIAN_POINT('Ctrl Pts',(2.4554069255945,14.3802831884086,2.33871751178352));
#455505=CARTESIAN_POINT('Ctrl Pts',(3.29905112134591,14.5385502142436,-0.784146194165878));
#455506=CARTESIAN_POINT('Ctrl Pts',(1.61181164346249,14.6622591874724,-2.66734747028903));
#455507=CARTESIAN_POINT('Ctrl Pts',(0.331201949128838,14.7332124854229,
-2.87133695619672));
#455508=CARTESIAN_POINT('Ctrl Pts',(0.00207587526855756,14.751410108095,
-2.8691175262514));
#455509=CARTESIAN_POINT('Ctrl Pts',(0.00201098180729838,13.948589891905,
-2.86897574933844));
#455510=CARTESIAN_POINT('Ctrl Pts',(-0.616636674456527,13.9827911062602,
-2.86494798953738));
#455511=CARTESIAN_POINT('Ctrl Pts',(-2.19548282131563,14.0697479958937,
-2.3654910683637));
#455512=CARTESIAN_POINT('Ctrl Pts',(-3.3830556511082,14.2094605608055,0.231430806858688));
#455513=CARTESIAN_POINT('Ctrl Pts',(-1.64968416256043,14.3677275866405,
2.96262862699381));
#455514=CARTESIAN_POINT('Ctrl Pts',(1.58493778894308,14.5259946124754,2.99776492739358));
#455515=CARTESIAN_POINT('Ctrl Pts',(3.37723035838085,14.6842616383104,0.304866953911748));
#455516=CARTESIAN_POINT('Ctrl Pts',(2.23702055240126,14.8251267314536,-2.33887228332351));
#455517=CARTESIAN_POINT('Ctrl Pts',(0.637020207330869,14.9132361493185,
-2.86482894038154));
#455518=CARTESIAN_POINT('Ctrl Pts',(-0.0022075361177263,14.948589891905,
-2.86945094346665));
#455519=CARTESIAN_POINT('Origin',(0.,5.25141010809499,0.));
#455520=CARTESIAN_POINT('',(-0.00245713763363008,12.751410108095,-2.87038222330126));
#455521=CARTESIAN_POINT('',(0.000575423425195377,12.948589891905,-2.87650911108102));
#455522=CARTESIAN_POINT('',(-1.47936051206424E-13,5.25141010809499,-2.872));
#455523=CARTESIAN_POINT('Ctrl Pts',(-0.00245713763363003,12.751410108095,
-2.87038222330126));
#455524=CARTESIAN_POINT('Ctrl Pts',(-0.280691862282867,12.7668110487496,
-2.87267579240923));
#455525=CARTESIAN_POINT('Ctrl Pts',(-1.50935892272592,12.8349676646826,
-2.70806675152048));
#455526=CARTESIAN_POINT('Ctrl Pts',(-3.25314999541872,12.9558799558939,
-0.956889911280283));
#455527=CARTESIAN_POINT('Ctrl Pts',(-2.5752272092837,13.1141469817289,2.20608885054153));
#455528=CARTESIAN_POINT('Ctrl Pts',(0.446212100842591,13.2724140075638,
3.36147556301922));
#455529=CARTESIAN_POINT('Ctrl Pts',(3.06158804260283,13.4306810333988,1.45784150227068));
#455530=CARTESIAN_POINT('Ctrl Pts',(2.89084781869623,13.5889480592338,-1.77246215397422));
#455531=CARTESIAN_POINT('Ctrl Pts',(0.998443281277944,13.6958577507992,
-2.86496636962172));
#455532=CARTESIAN_POINT('Ctrl Pts',(0.0255822995740321,13.7500117670862,
-2.87661661782493));
#455533=CARTESIAN_POINT('Ctrl Pts',(0.000460133735044324,13.751410108095,
-2.87656037903988));
#455534=CARTESIAN_POINT('Ctrl Pts',(0.00057542342519559,12.948589891905,
-2.87650911108102));
#455535=CARTESIAN_POINT('Ctrl Pts',(-0.915728012150204,12.9995903879236,
-2.87398439747242));
#455536=CARTESIAN_POINT('Ctrl Pts',(-2.78446322534953,13.1033465592205,
-1.90542149769778));
#455537=CARTESIAN_POINT('Ctrl Pts',(-3.14278767844486,13.2598584057957,
1.27338564834797));
#455538=CARTESIAN_POINT('Ctrl Pts',(-0.645120783207451,13.4181254316307,
3.32903057926365));
#455539=CARTESIAN_POINT('Ctrl Pts',(2.43962098791356,13.5763924574656,2.35518041283082));
#455540=CARTESIAN_POINT('Ctrl Pts',(3.30425105968087,13.7346594833006,-0.761938558424485));
#455541=CARTESIAN_POINT('Ctrl Pts',(1.62488632563581,13.8587252947804,-2.66191063110109));
#455542=CARTESIAN_POINT('Ctrl Pts',(0.337632800498971,13.9300354309819,
-2.87116084461198));
#455543=CARTESIAN_POINT('Ctrl Pts',(0.00201098180729838,13.948589891905,
-2.86897574933844));
#455544=CARTESIAN_POINT('Origin',(0.,5.25141010809499,0.));
#455545=CARTESIAN_POINT('',(0.00158946424445254,11.751410108095,-2.86827662802734));
#455546=CARTESIAN_POINT('',(-0.00248815572466116,11.948589891905,-2.87055996458015));
#455547=CARTESIAN_POINT('',(-1.47936051206424E-13,5.25141010809499,-2.872));
#455548=CARTESIAN_POINT('Ctrl Pts',(0.00158946424445229,11.751410108095,
-2.86827662802734));
#455549=CARTESIAN_POINT('Ctrl Pts',(-0.581219832021058,11.783610330413,
-2.86532506714357));
#455550=CARTESIAN_POINT('Ctrl Pts',(-2.12312024035974,11.8685662280094,
-2.41007181460196));
#455551=CARTESIAN_POINT('Ctrl Pts',(-3.38937612577637,12.0062778008841,
0.103695101446341));
#455552=CARTESIAN_POINT('Ctrl Pts',(-1.76022816749725,12.164544826719,2.89831330161118));
#455553=CARTESIAN_POINT('Ctrl Pts',(1.470768272467,12.322811852554,3.05539913673341));
#455554=CARTESIAN_POINT('Ctrl Pts',(3.36333145263819,12.481078878389,0.432000851345749));
#455555=CARTESIAN_POINT('Ctrl Pts',(2.30885711969421,12.6239449635693,-2.29099023912859));
#455556=CARTESIAN_POINT('Ctrl Pts',(0.67239672586907,12.7140553734713,-2.86481920820428));
#455557=CARTESIAN_POINT('Ctrl Pts',(-0.00245713763363003,12.751410108095,
-2.87038222330126));
#455558=CARTESIAN_POINT('Ctrl Pts',(-0.0024881557246614,11.948589891905,
-2.87055996458015));
#455559=CARTESIAN_POINT('Ctrl Pts',(-0.274233616854917,11.9636339943087,
-2.87283941429877));
#455560=CARTESIAN_POINT('Ctrl Pts',(-1.4962908949992,12.0314337719906,-2.71302462104432));
#455561=CARTESIAN_POINT('Ctrl Pts',(-3.24664049163476,12.1519892249509,
-0.978749670253043));
#455562=CARTESIAN_POINT('Ctrl Pts',(-2.59000777962451,12.3102562507859,
2.18871768405023));
#455563=CARTESIAN_POINT('Ctrl Pts',(0.423592117726756,12.4685232766209,
3.36440115286681));
#455564=CARTESIAN_POINT('Ctrl Pts',(3.05171335757124,12.6267903024558,1.47840149529983));
#455565=CARTESIAN_POINT('Ctrl Pts',(2.90270462181359,12.7850573282908,-1.75297783143327));
#455566=CARTESIAN_POINT('Ctrl Pts',(1.01139939624214,12.8923238581072,-2.86187502554507));
#455567=CARTESIAN_POINT('Ctrl Pts',(0.0321099556615316,12.9468347126453,
-2.87659599896072));
#455568=CARTESIAN_POINT('Ctrl Pts',(0.00057542342519559,12.948589891905,
-2.87650911108102));
#455569=CARTESIAN_POINT('Origin',(0.,5.25141010809499,0.));
#455570=CARTESIAN_POINT('',(0.00118908056354697,10.751410108095,-2.8760373750822));
#455571=CARTESIAN_POINT('',(0.00150509715381469,10.948589891905,-2.86817106627712));
#455572=CARTESIAN_POINT('',(-1.47936051206424E-13,5.25141010809499,-2.872));
#455573=CARTESIAN_POINT('Ctrl Pts',(0.00118908056354687,10.751410108095,
-2.8760373750822));
#455574=CARTESIAN_POINT('Ctrl Pts',(-0.87954819760536,10.8004096120764,
-2.87141110940037));
#455575=CARTESIAN_POINT('Ctrl Pts',(-2.71674168632202,10.9021647913362,
-1.96862591891224));
#455576=CARTESIAN_POINT('Ctrl Pts',(-3.18857005274037,11.0566756458742,
1.15396889840285));
#455577=CARTESIAN_POINT('Ctrl Pts',(-0.770195857929068,11.2149426717092,
3.30233576977685));
#455578=CARTESIAN_POINT('Ctrl Pts',(2.34907444021962,11.3732096975442,2.44550045375373));
#455579=CARTESIAN_POINT('Ctrl Pts',(3.33063248386109,11.5314767233792,-0.636797027311755));
#455580=CARTESIAN_POINT('Ctrl Pts',(1.69819735393824,11.6575435268961,-2.63038771649106));
#455581=CARTESIAN_POINT('Ctrl Pts',(0.373633761202303,11.7308546551347,
-2.87016079734477));
#455582=CARTESIAN_POINT('Ctrl Pts',(0.00158946424445229,11.751410108095,
-2.86827662802734));
#455583=CARTESIAN_POINT('Ctrl Pts',(0.00150509715381476,10.948589891905,
-2.86817106627712));
#455584=CARTESIAN_POINT('Ctrl Pts',(-0.574898968689857,10.980433275972,
-2.86541333431411));
#455585=CARTESIAN_POINT('Ctrl Pts',(-2.11018667018124,11.0650323353174,
-2.41780658533811));
#455586=CARTESIAN_POINT('Ctrl Pts',(-3.38999725238531,11.2023870699411,
0.0808951693976638));
#455587=CARTESIAN_POINT('Ctrl Pts',(-1.77968313098077,11.360654095776,2.88640838279897));
#455588=CARTESIAN_POINT('Ctrl Pts',(1.45018394022225,11.518921121611,3.06522298348167));
#455589=CARTESIAN_POINT('Ctrl Pts',(3.36034997176485,11.677188147446,0.454613535191446));
#455590=CARTESIAN_POINT('Ctrl Pts',(2.32162678658566,11.8204110708773,-2.28222762448876));
#455591=CARTESIAN_POINT('Ctrl Pts',(0.678705609501433,11.9108783190303,
-2.86484598897222));
#455592=CARTESIAN_POINT('Ctrl Pts',(-0.0024881557246614,11.948589891905,
-2.87055996458015));
#455593=CARTESIAN_POINT('Origin',(0.,5.25141010809499,0.));
#455594=CARTESIAN_POINT('',(-0.00258136649849588,9.75141010809498,-2.87160024361889));
#455595=CARTESIAN_POINT('',(0.00129076080759852,9.94858989190502,-2.87592458636046));
#455596=CARTESIAN_POINT('',(-1.47936051206424E-13,5.25141010809499,-2.872));
#455597=CARTESIAN_POINT('Ctrl Pts',(-0.00258136649849569,9.75141010809498,
-2.87160024361889));
#455598=CARTESIAN_POINT('Ctrl Pts',(-0.237965141875198,9.76445321846148,
-2.87371275150489));
#455599=CARTESIAN_POINT('Ctrl Pts',(-1.42303883068652,9.8302520041063,-2.73984855250909));
#455600=CARTESIAN_POINT('Ctrl Pts',(-3.20742346381156,9.94880646502946,
-1.10048057409996));
#455601=CARTESIAN_POINT('Ctrl Pts',(-2.67069952678566,10.1070734908644,
2.08949452686489));
#455602=CARTESIAN_POINT('Ctrl Pts',(0.29642307182911,10.2653405166994,3.3779811414132));
#455603=CARTESIAN_POINT('Ctrl Pts',(2.99379373691612,10.4236075425344,1.59242651290754));
#455604=CARTESIAN_POINT('Ctrl Pts',(2.96674265574526,10.5818745683693,-1.64227319112547));
#455605=CARTESIAN_POINT('Ctrl Pts',(1.08412200216352,10.6911420902229,-2.84370207199545));
#455606=CARTESIAN_POINT('Ctrl Pts',(0.0687040514418887,10.7476539367981,
-2.87639201227143));
#455607=CARTESIAN_POINT('Ctrl Pts',(0.00118908056354687,10.751410108095,
-2.8760373750822));
#455608=CARTESIAN_POINT('Ctrl Pts',(0.0012907608075984,9.94858989190502,
-2.87592458636046));
#455609=CARTESIAN_POINT('Ctrl Pts',(-0.873123805142145,9.99723255763544,
-2.87100311148923));
#455610=CARTESIAN_POINT('Ctrl Pts',(-2.70457728265256,10.0986308986442,
-1.97965085114474));
#455611=CARTESIAN_POINT('Ctrl Pts',(-3.19626004985765,10.2527849149312,
1.13249596744652));
#455612=CARTESIAN_POINT('Ctrl Pts',(-0.792390653220595,10.4110519407662,
3.29708089890013));
#455613=CARTESIAN_POINT('Ctrl Pts',(2.33257261886262,10.5693189666012,2.46124569460491));
#455614=CARTESIAN_POINT('Ctrl Pts',(3.33484068029608,10.7275859924362,-0.614380207850174));
#455615=CARTESIAN_POINT('Ctrl Pts',(1.71126896779768,10.8540096342041,-2.62457997243907));
#455616=CARTESIAN_POINT('Ctrl Pts',(0.380043058286468,10.9276776006937,
-2.86998213302089));
#455617=CARTESIAN_POINT('Ctrl Pts',(0.00150509715381476,10.948589891905,
-2.86817106627712));
#455618=CARTESIAN_POINT('Origin',(0.,5.25141010809499,0.));
#455619=CARTESIAN_POINT('',(0.000993903865917874,8.75141010809498,-2.86769215449362));
#455620=CARTESIAN_POINT('',(-0.00258314593131442,8.94858989190502,-2.87179187325464));
#455621=CARTESIAN_POINT('',(-1.47936051206424E-13,5.25141010809499,-2.872));
#455622=CARTESIAN_POINT('Ctrl Pts',(0.000993903865917981,8.75141010809497,
-2.86769215449362));
#455623=CARTESIAN_POINT('Ctrl Pts',(-0.539416506838244,8.78125250012487,
-2.86600725099512));
#455624=CARTESIAN_POINT('Ctrl Pts',(-2.0375213686481,8.8638505674331,-2.45998816760348));
#455625=CARTESIAN_POINT('Ctrl Pts',(-3.39063316576441,8.99920431001964,
-0.0469946717703988));
#455626=CARTESIAN_POINT('Ctrl Pts',(-1.88726201450869,9.1574713358546,2.81724502982847));
#455627=CARTESIAN_POINT('Ctrl Pts',(1.33356715403539,9.31573836168959,3.11772757096118));
#455628=CARTESIAN_POINT('Ctrl Pts',(3.34081625807316,9.47400538752454,0.581005048681307));
#455629=CARTESIAN_POINT('Ctrl Pts',(2.392975748847,9.61922930299303,-2.23181518064891));
#455630=CARTESIAN_POINT('Ctrl Pts',(0.714095346047257,9.71169754318316,
-2.86516825736777));
#455631=CARTESIAN_POINT('Ctrl Pts',(-0.00258136649849569,9.75141010809498,
-2.87160024361889));
#455632=CARTESIAN_POINT('Ctrl Pts',(-0.00258314593131425,8.94858989190502,
-2.87179187325464));
#455633=CARTESIAN_POINT('Ctrl Pts',(-0.231488332032663,8.96127616402051,
-2.87386034028333));
#455634=CARTESIAN_POINT('Ctrl Pts',(-1.40998235584436,9.02671811141432,
-2.7444605327945));
#455635=CARTESIAN_POINT('Ctrl Pts',(-3.19994881461505,9.14491573408647,
-1.12202938400675));
#455636=CARTESIAN_POINT('Ctrl Pts',(-2.68469389625817,9.30318275992144,
2.07148374386093));
#455637=CARTESIAN_POINT('Ctrl Pts',(0.273695539681721,9.4614497857564,3.37989889026531));
#455638=CARTESIAN_POINT('Ctrl Pts',(2.98301528359298,9.61971681159137,1.61252745511383));
#455639=CARTESIAN_POINT('Ctrl Pts',(2.97772210058549,9.77798383742635,-1.62228130541839));
#455640=CARTESIAN_POINT('Ctrl Pts',(1.09710326595299,9.88760819753089,-2.8403108118492));
#455641=CARTESIAN_POINT('Ctrl Pts',(0.0752274047922757,9.94447688235712,
-2.87634072459695));
#455642=CARTESIAN_POINT('Ctrl Pts',(0.0012907608075984,9.94858989190502,
-2.87592458636046));
#455643=CARTESIAN_POINT('Origin',(0.,5.25141010809499,0.));
#455644=CARTESIAN_POINT('',(0.00198847260380099,7.75141010809497,-2.87512062938712));
#455645=CARTESIAN_POINT('',(0.000911915543898995,7.94858989190502,-2.86762206492074));
#455646=CARTESIAN_POINT('',(-1.47936051206424E-13,5.25141010809499,-2.872));
#455647=CARTESIAN_POINT('Ctrl Pts',(0.00198847260380112,7.75141010809497,
-2.87512062938712));
#455648=CARTESIAN_POINT('Ctrl Pts',(-0.837002867190702,7.79805178178826,
-2.86893764875045));
#455649=CARTESIAN_POINT('Ctrl Pts',(-2.63619448267628,7.89744913075989,
-2.04016147455094));
#455650=CARTESIAN_POINT('Ctrl Pts',(-3.23653135410128,8.0496021550098,1.01119616857442));
#455651=CARTESIAN_POINT('Ctrl Pts',(-0.91623943503461,8.2078691808448,3.26483823460727));
#455652=CARTESIAN_POINT('Ctrl Pts',(2.23814586565504,8.36613620667974,2.54746254727596));
#455653=CARTESIAN_POINT('Ctrl Pts',(3.355613622894,8.52440323251474,-0.488194768594614));
#455654=CARTESIAN_POINT('Ctrl Pts',(1.78454755545998,8.6528278663198,-2.59094511229407));
#455655=CARTESIAN_POINT('Ctrl Pts',(0.415926352928926,8.72849682484655,
-2.86898584003561));
#455656=CARTESIAN_POINT('Ctrl Pts',(0.000993903865917981,8.75141010809497,
-2.86769215449362));
#455657=CARTESIAN_POINT('Ctrl Pts',(0.000911915543898995,7.94858989190502,
-2.86762206492074));
#455658=CARTESIAN_POINT('Ctrl Pts',(-0.533073886542687,7.9780754456839,
-2.86612649557932));
#455659=CARTESIAN_POINT('Ctrl Pts',(-2.02456627808555,8.06031667474111,
-2.46731154287715));
#455660=CARTESIAN_POINT('Ctrl Pts',(-3.39022251156056,8.19531357907665,
-0.0697920698937834));
#455661=CARTESIAN_POINT('Ctrl Pts',(-1.90617827987364,8.3535806049116,2.80448353848272));
#455662=CARTESIAN_POINT('Ctrl Pts',(1.31257158419998,8.5118476307466,3.12662922130667));
#455663=CARTESIAN_POINT('Ctrl Pts',(3.33683050597697,8.67011465658154,0.603461870573552));
#455664=CARTESIAN_POINT('Ctrl Pts',(2.40565202370955,8.81569541030104,-2.22259592592606));
#455665=CARTESIAN_POINT('Ctrl Pts',(0.720410504564146,8.90852048874219,
-2.86525865068561));
#455666=CARTESIAN_POINT('Ctrl Pts',(-0.00258314593131425,8.94858989190502,
-2.87179187325464));
#455667=CARTESIAN_POINT('Origin',(0.,0.,0.));
#455668=CARTESIAN_POINT('',(0.00234742734116236,0.322176117089595,-2.94408456759461));
#455669=CARTESIAN_POINT('',(0.00309359675299801,0.177823882910405,-2.94421791268484));
#455670=CARTESIAN_POINT('',(-3.60291088309151E-16,0.,-2.942));
#455671=CARTESIAN_POINT('',(2.64462557919718,0.,1.28892185405323));
#455672=CARTESIAN_POINT('Ctrl Pts',(0.00234742734116236,0.322176117089595,
-2.94408456759461));
#455673=CARTESIAN_POINT('Ctrl Pts',(0.152623335834112,0.31402898266599,
-2.94532683936105));
#455674=CARTESIAN_POINT('Ctrl Pts',(0.302716573408032,0.305881848242384,
-2.93478849511196));
#455675=CARTESIAN_POINT('Ctrl Pts',(0.450880220883188,0.297734713818779,
-2.9118552212362));
#455676=CARTESIAN_POINT('Ctrl Pts',(1.40105040066211,0.245487321750099,
-2.76478464533735));
#455677=CARTESIAN_POINT('Ctrl Pts',(2.27186370990282,0.193239929681419,
-2.10795667259909));
#455678=CARTESIAN_POINT('Ctrl Pts',(2.67509378307532,0.140992537612738,
-1.23478030777358));
#455679=CARTESIAN_POINT('Ctrl Pts',(3.0378068232696,0.0939950250751588,
-0.449341733165658));
#455680=CARTESIAN_POINT('Ctrl Pts',(3.02218231782814,0.0469975125375793,
0.511151705155529));
#455681=CARTESIAN_POINT('Ctrl Pts',(2.64767078191736,-2.62376925741492E-16,
1.2919591116057));
#455682=CARTESIAN_POINT('',(2.64462557919717,0.,-1.28892185405323));
#455683=CARTESIAN_POINT('Origin',(0.,0.,0.));
#455684=CARTESIAN_POINT('Ctrl Pts',(2.64462557919718,0.,-1.28892185405323));
#455685=CARTESIAN_POINT('Ctrl Pts',(2.22149825342052,0.0522473920686802,
-2.15709966133247));
#455686=CARTESIAN_POINT('Ctrl Pts',(1.34158650816433,0.104494784137361,
-2.79385315646035));
#455687=CARTESIAN_POINT('Ctrl Pts',(0.389878440861619,0.156742176206041,
-2.92042183738268));
#455688=CARTESIAN_POINT('Ctrl Pts',(0.26187441011064,0.163769411774162,
-2.93744523130095));
#455689=CARTESIAN_POINT('Ctrl Pts',(0.132571580237253,0.170796647342284,
-2.94523935594652));
#455690=CARTESIAN_POINT('Ctrl Pts',(0.00309359675299801,0.177823882910405,
-2.94421791268484));
#455691=CARTESIAN_POINT('Origin',(0.,0.,0.));
#455692=CARTESIAN_POINT('',(-0.000533914549282755,1.3221761170896,-2.93754474843028));
#455693=CARTESIAN_POINT('',(-0.000201976967395493,1.1778238829104,-2.93745911239609));
#455694=CARTESIAN_POINT('',(-3.60291088309151E-16,0.,-2.942));
#455695=CARTESIAN_POINT('Ctrl Pts',(-0.000533914549282755,1.3221761170896,
-2.93754474843028));
#455696=CARTESIAN_POINT('Ctrl Pts',(0.518827038902267,1.29418000174474,
-2.93667747579154));
#455697=CARTESIAN_POINT('Ctrl Pts',(1.03859776609672,1.26618388639988,-2.80518365811747));
#455698=CARTESIAN_POINT('Ctrl Pts',(1.48377366790336,1.23818777105502,-2.54571195061657));
#455699=CARTESIAN_POINT('Ctrl Pts',(2.31457749888888,1.18594037898634,-2.06147619627931));
#455700=CARTESIAN_POINT('Ctrl Pts',(2.8855793906847,1.13369298691766,-1.13151376080079));
#455701=CARTESIAN_POINT('Ctrl Pts',(2.94155991415087,1.08144559484898,-0.171517343472406));
#455702=CARTESIAN_POINT('Ctrl Pts',(2.99754043761704,1.0291982027803,0.788479073855973));
#455703=CARTESIAN_POINT('Ctrl Pts',(2.53849959275358,0.976950810711622,
1.77850947303422));
#455704=CARTESIAN_POINT('Ctrl Pts',(1.7695909716078,0.924703418642942,2.35601906999579));
#455705=CARTESIAN_POINT('Ctrl Pts',(1.00068235046202,0.872456026574262,
2.93352866695737));
#455706=CARTESIAN_POINT('Ctrl Pts',(-0.0780940469660901,0.820208634505582,
3.09851746170227));
#455707=CARTESIAN_POINT('Ctrl Pts',(-0.984445713078919,0.767961242436901,
2.77724933044992));
#455708=CARTESIAN_POINT('Ctrl Pts',(-1.89079737919174,0.715713850368221,
2.45598119919756));
#455709=CARTESIAN_POINT('Ctrl Pts',(-2.62472431398929,0.66346645829954,
1.64845614194797));
#455710=CARTESIAN_POINT('Ctrl Pts',(-2.85830324984526,0.61121906623086,
0.715613073331115));
#455711=CARTESIAN_POINT('Ctrl Pts',(-3.09188218570122,0.55897167416218,
-0.217229995285738));
#455712=CARTESIAN_POINT('Ctrl Pts',(-2.8251131226156,0.5067242820935,-1.27539107526984));
#455713=CARTESIAN_POINT('Ctrl Pts',(-2.17696506591423,0.45447689002482,
-1.98581502573217));
#455714=CARTESIAN_POINT('Ctrl Pts',(-1.62988519913137,0.410376632379746,
-2.58545986946785));
#455715=CARTESIAN_POINT('Ctrl Pts',(-0.811092726927701,0.36627637473467,
-2.93736017812011));
#455716=CARTESIAN_POINT('Ctrl Pts',(0.00234742734116236,0.322176117089595,
-2.94408456759461));
#455717=CARTESIAN_POINT('Ctrl Pts',(0.00309359675299801,0.177823882910405,
-2.94421791268484));
#455718=CARTESIAN_POINT('Ctrl Pts',(-0.830095303743749,0.223044039410964,
-2.93764494046812));
#455719=CARTESIAN_POINT('Ctrl Pts',(-1.67053714603895,0.268264195911523,
-2.56602781851946));
#455720=CARTESIAN_POINT('Ctrl Pts',(-2.2188180236089,0.313484352412081,
-1.93960410903164));
#455721=CARTESIAN_POINT('Ctrl Pts',(-2.85230203142748,0.365731744480761,
-1.2158338330415));
#455722=CARTESIAN_POINT('Ctrl Pts',(-3.09576565771542,0.417979136549442,
-0.151909414344424));
#455723=CARTESIAN_POINT('Ctrl Pts',(-2.84232694733696,0.470226528618122,
0.775884131996558));
#455724=CARTESIAN_POINT('Ctrl Pts',(-2.5888882369585,0.522473920686802,
1.70367767833754));
#455725=CARTESIAN_POINT('Ctrl Pts',(-1.83854718991364,0.574721312755483,
2.49534035232244));
#455726=CARTESIAN_POINT('Ctrl Pts',(-0.925728335606107,0.626968704824163,
2.79735991175273));
#455727=CARTESIAN_POINT('Ctrl Pts',(-0.0129094812985767,0.679216096892843,
3.09937947118302));
#455728=CARTESIAN_POINT('Ctrl Pts',(1.06238718027163,0.731463488961522,
2.91175591605871));
#455729=CARTESIAN_POINT('Ctrl Pts',(1.8189927749781,0.783710881030203,2.31816853201152));
#455730=CARTESIAN_POINT('Ctrl Pts',(2.57559836968458,0.835958273098883,
1.72458114796434));
#455731=CARTESIAN_POINT('Ctrl Pts',(3.01351289752732,0.888205665167564,
0.725029934994281));
#455732=CARTESIAN_POINT('Ctrl Pts',(2.93725089347923,0.940453057236245,
-0.233583529514978));
#455733=CARTESIAN_POINT('Ctrl Pts',(2.86098888943113,0.992700449304925,
-1.19219699402423));
#455734=CARTESIAN_POINT('Ctrl Pts',(2.2705503534922,1.0449478413736,-2.10987271007269));
#455735=CARTESIAN_POINT('Ctrl Pts',(1.42972599524097,1.09719523344228,-2.57645757349211));
#455736=CARTESIAN_POINT('Ctrl Pts',(0.99720340249237,1.12407144993166,-2.81647023830494));
#455737=CARTESIAN_POINT('Ctrl Pts',(0.498426099280125,1.15094766642103,
-2.93711953997791));
#455738=CARTESIAN_POINT('Ctrl Pts',(-0.000201976967395493,1.1778238829104,
-2.93745911239609));
#455739=CARTESIAN_POINT('Origin',(0.,0.,0.));
#455740=CARTESIAN_POINT('',(-0.00134644729286121,2.3221761170896,-2.94573633641246));
#455741=CARTESIAN_POINT('',(-0.00163187090823506,2.1778238829104,-2.94531716671524));
#455742=CARTESIAN_POINT('',(-3.60291088309151E-16,0.,-2.942));
#455743=CARTESIAN_POINT('Ctrl Pts',(-0.00134644729286121,2.3221761170896,
-2.94573633641246));
#455744=CARTESIAN_POINT('Ctrl Pts',(0.879913779079956,2.27433102082349,
-2.94064754527962));
#455745=CARTESIAN_POINT('Ctrl Pts',(1.7654150896307,2.22648592455738,-2.51813317797539));
#455746=CARTESIAN_POINT('Ctrl Pts',(2.31152197537838,2.17864082829127,-1.82731873918827));
#455747=CARTESIAN_POINT('Ctrl Pts',(2.90787693749131,2.12639343622259,-1.07294147491715));
#455748=CARTESIAN_POINT('Ctrl Pts',(3.09950779265045,2.07414604415391,0.00138066437529602));
#455749=CARTESIAN_POINT('Ctrl Pts',(2.80075519910971,2.02189865208523,0.915421823845812));
#455750=CARTESIAN_POINT('Ctrl Pts',(2.50200260556897,1.96965126001655,1.82946298331634));
#455751=CARTESIAN_POINT('Ctrl Pts',(1.71286656332835,1.91740386794787,2.58322316296495));
#455752=CARTESIAN_POINT('Ctrl Pts',(0.786093029068817,1.86515647587919,
2.83976862276147));
#455753=CARTESIAN_POINT('Ctrl Pts',(-0.140680505190703,1.81290908381051,
3.09631408255799));
#455754=CARTESIAN_POINT('Ctrl Pts',(-1.20509153146913,1.76066169174183,
2.85564482250244));
#455755=CARTESIAN_POINT('Ctrl Pts',(-1.93134289750084,1.70841429967315,
2.22534118511019));
#455756=CARTESIAN_POINT('Ctrl Pts',(-2.65759426353255,1.65616690760447,
1.59503754771794));
#455757=CARTESIAN_POINT('Ctrl Pts',(-3.04568596931755,1.60391951553579,
0.575099532988995));
#455758=CARTESIAN_POINT('Ctrl Pts',(-2.92214249359839,1.55167212346711,
-0.378557369309796));
#455759=CARTESIAN_POINT('Ctrl Pts',(-2.79859901787924,1.49942473139842,
-1.33221427160858));
#455760=CARTESIAN_POINT('Ctrl Pts',(-2.16342036065593,1.44717733932974,
-2.21959006147722));
#455761=CARTESIAN_POINT('Ctrl Pts',(-1.30052814695666,1.39492994726106,
-2.64402341981353));
#455762=CARTESIAN_POINT('Ctrl Pts',(-0.900005995922876,1.37067867053724,
-2.84102944090459));
#455763=CARTESIAN_POINT('Ctrl Pts',(-0.450423695561913,1.34642739381342,
-2.93829601225735));
#455764=CARTESIAN_POINT('Ctrl Pts',(-0.000533914549282755,1.3221761170896,
-2.93754474843028));
#455765=CARTESIAN_POINT('Ctrl Pts',(-0.000201976967395493,1.1778238829104,
-2.93745911239609));
#455766=CARTESIAN_POINT('Ctrl Pts',(-0.470907385827677,1.20319505848971,
-2.93777966910268));
#455767=CARTESIAN_POINT('Ctrl Pts',(-0.941479812882249,1.22856623406902,
-2.83088766492598));
#455768=CARTESIAN_POINT('Ctrl Pts',(-1.35605793578947,1.25393740964832,
-2.61598698348122));
#455769=CARTESIAN_POINT('Ctrl Pts',(-2.20980732800516,1.30618480171701,
-2.17343751926055));
#455770=CARTESIAN_POINT('Ctrl Pts',(-2.82609593187302,1.35843219378569,
-1.27284458002884));
#455771=CARTESIAN_POINT('Ctrl Pts',(-2.92947779976765,1.41067958585437,
-0.31679046293656));
#455772=CARTESIAN_POINT('Ctrl Pts',(-3.03285966766227,1.46292697792305,
0.639263654155722));
#455773=CARTESIAN_POINT('Ctrl Pts',(-2.62333479958367,1.51517436999173,
1.65077894910857));
#455774=CARTESIAN_POINT('Ctrl Pts',(-1.88394286986409,1.56742176206041,
2.2656116195793));
#455775=CARTESIAN_POINT('Ctrl Pts',(-1.14455094014452,1.61966915412909,
2.88044429005002));
#455776=CARTESIAN_POINT('Ctrl Pts',(-0.0752919487839852,1.67191654619777,
3.09859433603862));
#455777=CARTESIAN_POINT('Ctrl Pts',(0.845861261610144,1.72416393826645,
2.82254409907328));
#455778=CARTESIAN_POINT('Ctrl Pts',(1.76701447200428,1.77641133033513,2.54649386210794));
#455779=CARTESIAN_POINT('Ctrl Pts',(2.54006190143201,1.82865872240381,1.77624334218867));
#455780=CARTESIAN_POINT('Ctrl Pts',(2.81945377803531,1.88090611447249,0.856099332179975));
#455781=CARTESIAN_POINT('Ctrl Pts',(3.09884565463862,1.93315350654117,-0.0640446778287201));
#455782=CARTESIAN_POINT('Ctrl Pts',(2.88458197841751,1.98540089860985,-1.13408217792684));
#455783=CARTESIAN_POINT('Ctrl Pts',(2.2724366580869,2.03764829067853,-1.87570349193988));
#455784=CARTESIAN_POINT('Ctrl Pts',(1.72499094254115,2.08437348808915,-2.53894046758902));
#455785=CARTESIAN_POINT('Ctrl Pts',(0.859325602669026,2.13109868549978,
-2.93951522469678));
#455786=CARTESIAN_POINT('Ctrl Pts',(-0.00163187090823506,2.1778238829104,
-2.94531716671524));
#455787=CARTESIAN_POINT('Origin',(0.,0.,0.));
#455788=CARTESIAN_POINT('',(0.00237334009290435,3.3221761170896,-2.94031398119338));
#455789=CARTESIAN_POINT('',(0.00246242204629553,3.1778238829104,-2.94087084915089));
#455790=CARTESIAN_POINT('',(-3.60291088309151E-16,0.,-2.942));
#455791=CARTESIAN_POINT('Ctrl Pts',(0.00237334009290435,3.3221761170896,
-2.94031398119338));
#455792=CARTESIAN_POINT('Ctrl Pts',(0.288247022003705,3.30672943197091,
-2.94257327477183));
#455793=CARTESIAN_POINT('Ctrl Pts',(0.573526739760804,3.29128274685223,
-2.90415646478538));
#455794=CARTESIAN_POINT('Ctrl Pts',(0.845861119733735,3.27583606173355,
-2.82254358189058));
#455795=CARTESIAN_POINT('Ctrl Pts',(1.76701417068956,3.22358866966487,-2.54649339651438));
#455796=CARTESIAN_POINT('Ctrl Pts',(2.54006143235309,3.17134127759619,-1.77624301496856));
#455797=CARTESIAN_POINT('Ctrl Pts',(2.81945325191896,3.11909388552751,-0.856099173574967));
#455798=CARTESIAN_POINT('Ctrl Pts',(3.09884507148485,3.06684649345883,0.06404466781863));
#455799=CARTESIAN_POINT('Ctrl Pts',(2.88458144895307,3.01459910139015,1.13408196906));
#455800=CARTESIAN_POINT('Ctrl Pts',(2.27243624440142,2.96235170932147,1.87570314629083));
#455801=CARTESIAN_POINT('Ctrl Pts',(1.66029103984977,2.91010431725279,2.61732432352167));
#455802=CARTESIAN_POINT('Ctrl Pts',(0.650264253278263,2.85785692518411,
3.03052937674198));
#455803=CARTESIAN_POINT('Ctrl Pts',(-0.306156988195277,2.80560953311543,
2.93061358417489));
#455804=CARTESIAN_POINT('Ctrl Pts',(-1.26257822966882,2.75336214104675,
2.8306977916078));
#455805=CARTESIAN_POINT('Ctrl Pts',(-2.16539392604439,2.70111474897807,
2.21766115325329));
#455806=CARTESIAN_POINT('Ctrl Pts',(-2.61104285907814,2.64886735690939,
1.36553359130061));
#455807=CARTESIAN_POINT('Ctrl Pts',(-3.05669179211189,2.59661996484071,
0.51340602934793));
#455808=CARTESIAN_POINT('Ctrl Pts',(-3.04517396180382,2.54437257277203,
-0.577812456202931));
#455809=CARTESIAN_POINT('Ctrl Pts',(-2.58163754554515,2.49212518070335,
-1.42034333901256));
#455810=CARTESIAN_POINT('Ctrl Pts',(-2.11810112928649,2.43987778863467,
-2.26287422182219));
#455811=CARTESIAN_POINT('Ctrl Pts',(-1.20254612707725,2.38763039656599,
-2.85671750189059));
#455812=CARTESIAN_POINT('Ctrl Pts',(-0.244229091439268,2.33538300449731,
-2.93642294729989));
#455813=CARTESIAN_POINT('Ctrl Pts',(-0.163482571919671,2.33098070869474,
-2.9431388221766));
#455814=CARTESIAN_POINT('Ctrl Pts',(-0.0824324623351636,2.32657841289217,
-2.94620456336972));
#455815=CARTESIAN_POINT('Ctrl Pts',(-0.00134644729286121,2.3221761170896,
-2.94573633641246));
#455816=CARTESIAN_POINT('Ctrl Pts',(-0.00163187090823506,2.1778238829104,
-2.94531716671524));
#455817=CARTESIAN_POINT('Ctrl Pts',(-0.103383709848986,2.18334607756846,
-2.94600286640184));
#455818=CARTESIAN_POINT('Ctrl Pts',(-0.205069791295828,2.18886827222651,
-2.94117454564737));
#455819=CARTESIAN_POINT('Ctrl Pts',(-0.306157042210219,2.19439046688457,
-2.93061412268682));
#455820=CARTESIAN_POINT('Ctrl Pts',(-1.26257845773664,2.24663785895325,
-2.83069831149277));
#455821=CARTESIAN_POINT('Ctrl Pts',(-2.16539432434938,2.29888525102193,
-2.2176615611767));
#455822=CARTESIAN_POINT('Ctrl Pts',(-2.6110433404237,2.35113264309061,-1.36553384267249));
#455823=CARTESIAN_POINT('Ctrl Pts',(-3.05669235649802,2.40338003515929,
-0.513406124168287));
#455824=CARTESIAN_POINT('Ctrl Pts',(-3.04517452203392,2.45562742722797,
0.577812562524056));
#455825=CARTESIAN_POINT('Ctrl Pts',(-2.58163801980982,2.50787481929665,
1.42034360036398));
#455826=CARTESIAN_POINT('Ctrl Pts',(-2.11810151758573,2.56012221136533,
2.2628746382039));
#455827=CARTESIAN_POINT('Ctrl Pts',(-1.20254634760163,2.61236960343401,
2.8567180271914));
#455828=CARTESIAN_POINT('Ctrl Pts',(-0.244229136344604,2.66461699550269,
2.93642348720734));
#455829=CARTESIAN_POINT('Ctrl Pts',(0.714088074912416,2.71686438757137,
3.01612894722328));
#455830=CARTESIAN_POINT('Ctrl Pts',(1.71516732744236,2.76911177964005,2.58169647826766));
#455831=CARTESIAN_POINT('Ctrl Pts',(2.31152239995082,2.82135917170873,1.82731907529804));
#455832=CARTESIAN_POINT('Ctrl Pts',(2.90787747245929,2.87360656377741,1.07294167232842));
#455833=CARTESIAN_POINT('Ctrl Pts',(3.09950836494629,2.92585395584609,-0.00138066465518699));
#455834=CARTESIAN_POINT('Ctrl Pts',(2.80075571536857,2.97810134791477,-0.915421992244635));
#455835=CARTESIAN_POINT('Ctrl Pts',(2.50200306579085,3.03034873998345,-1.82946331983409));
#455836=CARTESIAN_POINT('Ctrl Pts',(1.71286687414841,3.08259613205213,-2.58322363802937));
#455837=CARTESIAN_POINT('Ctrl Pts',(0.786093171304736,3.13484352412081,
-2.83976914495077));
#455838=CARTESIAN_POINT('Ctrl Pts',(0.531962041897567,3.14917031038401,
-2.91011663023032));
#455839=CARTESIAN_POINT('Ctrl Pts',(0.26748175157528,3.16349709664721,-2.94307782418315));
#455840=CARTESIAN_POINT('Ctrl Pts',(0.00246242204629553,3.1778238829104,
-2.94087084915089));
#455841=CARTESIAN_POINT('Origin',(0.,0.,0.));
#455842=CARTESIAN_POINT('',(-0.00235626413880502,4.3221761170896,-2.93955723260335));
#455843=CARTESIAN_POINT('',(-0.00203590851197863,4.17782388291041,-2.93914442058615));
#455844=CARTESIAN_POINT('',(-3.60291088309151E-16,0.,-2.942));
#455845=CARTESIAN_POINT('Ctrl Pts',(-0.00235626413880502,4.3221761170896,
-2.93955723260335));
#455846=CARTESIAN_POINT('Ctrl Pts',(0.651304352142019,4.28688045104966,
-2.93489446451832));
#455847=CARTESIAN_POINT('Ctrl Pts',(1.30786871926028,4.25158478500973,-2.71916533387861));
#455848=CARTESIAN_POINT('Ctrl Pts',(1.81899283066209,4.2162891189698,-2.31816809067732));
#455849=CARTESIAN_POINT('Ctrl Pts',(2.57559852309904,4.16404172690112,-1.72458076014517));
#455850=CARTESIAN_POINT('Ctrl Pts',(3.01351225985306,4.11179433483244,-0.725029779266838));
#455851=CARTESIAN_POINT('Ctrl Pts',(2.93725012432094,4.05954694276376,0.233583488232732));
#455852=CARTESIAN_POINT('Ctrl Pts',(2.86098798878882,4.00729955069508,1.1921967557323));
#455853=CARTESIAN_POINT('Ctrl Pts',(2.27054998097057,3.9550521586264,2.10987230985309));
#455854=CARTESIAN_POINT('Ctrl Pts',(1.42972586492197,3.90280476655772,2.57645709389019));
#455855=CARTESIAN_POINT('Ctrl Pts',(0.588901748873358,3.85055737448904,
3.0430418779273));
#455856=CARTESIAN_POINT('Ctrl Pts',(-0.502308475405612,3.79830998242035,
3.05853589188072));
#455857=CARTESIAN_POINT('Ctrl Pts',(-1.35605776241588,3.74606259035167,
2.61598650798725));
#455858=CARTESIAN_POINT('Ctrl Pts',(-2.20980704942615,3.69381519828299,
2.17343712409378));
#455859=CARTESIAN_POINT('Ctrl Pts',(-2.82609539916772,3.64156780621432,
1.27284434235344));
#455860=CARTESIAN_POINT('Ctrl Pts',(-2.92947721784002,3.58932041414564,
0.316790400434435));
#455861=CARTESIAN_POINT('Ctrl Pts',(-3.03285903651231,3.53707302207696,
-0.639263541484576));
#455862=CARTESIAN_POINT('Ctrl Pts',(-2.62333432411533,3.48482563000827,
-1.65077864358225));
#455863=CARTESIAN_POINT('Ctrl Pts',(-1.88394254779278,3.43257823793959,
-2.26561120002781));
#455864=CARTESIAN_POINT('Ctrl Pts',(-1.36314832239072,3.39577753098959,
-2.69867152777258));
#455865=CARTESIAN_POINT('Ctrl Pts',(-0.678701823405697,3.35897682403959,
-2.93493136348248));
#455866=CARTESIAN_POINT('Ctrl Pts',(0.00237334009290435,3.3221761170896,
-2.94031398119338));
#455867=CARTESIAN_POINT('Ctrl Pts',(0.00246242204629553,3.1778238829104,
-2.94087084915089));
#455868=CARTESIAN_POINT('Ctrl Pts',(-0.698999395089763,3.21574448871589,
-2.93502935555397));
#455869=CARTESIAN_POINT('Ctrl Pts',(-1.40423757166641,3.25366509452137,
-2.68280940691118));
#455870=CARTESIAN_POINT('Ctrl Pts',(-1.93134324840035,3.29158570032686,
-2.22534159435153));
#455871=CARTESIAN_POINT('Ctrl Pts',(-2.65759475121686,3.34383309239554,
-1.59503784118338));
#455872=CARTESIAN_POINT('Ctrl Pts',(-3.04568654280498,3.39608048446422,
-0.575099639199598));
#455873=CARTESIAN_POINT('Ctrl Pts',(-2.92214303868762,3.4483278765329,0.378557438820167));
#455874=CARTESIAN_POINT('Ctrl Pts',(-2.79859953457026,3.50057526860158,
1.33221451683994));
#455875=CARTESIAN_POINT('Ctrl Pts',(-2.16342073474742,3.55282266067026,
2.21959047089569));
#455876=CARTESIAN_POINT('Ctrl Pts',(-1.30052837232317,3.60507005273893,
2.64402390645178));
#455877=CARTESIAN_POINT('Ctrl Pts',(-0.437636009898931,3.65731744480762,
3.06845734200787));
#455878=CARTESIAN_POINT('Ctrl Pts',(0.652969915126714,3.7095648368763,3.02994825906432));
#455879=CARTESIAN_POINT('Ctrl Pts',(1.48377391623871,3.76181222894498,2.54571241761008));
#455880=CARTESIAN_POINT('Ctrl Pts',(2.3145779173507,3.81405962101366,2.06147657615583));
#455881=CARTESIAN_POINT('Ctrl Pts',(2.88557999454904,3.86630701308234,1.13151397619092));
#455882=CARTESIAN_POINT('Ctrl Pts',(2.94156049840815,3.91855440515102,0.171517377964578));
#455883=CARTESIAN_POINT('Ctrl Pts',(2.99754100226726,3.9708017972197,-0.788479220261775));
#455884=CARTESIAN_POINT('Ctrl Pts',(2.53849993278712,4.02304918928838,-1.77850981674955));
#455885=CARTESIAN_POINT('Ctrl Pts',(1.76959122115166,4.07529658135706,-2.35601951031475));
#455886=CARTESIAN_POINT('Ctrl Pts',(1.2666370243105,4.10947234854151,-2.7337768691529));
#455887=CARTESIAN_POINT('Ctrl Pts',(0.631101141471884,4.14364811572596,
-2.93503074915652));
#455888=CARTESIAN_POINT('Ctrl Pts',(-0.00203590851197863,4.17782388291041,
-2.93914442058615));
#455889=CARTESIAN_POINT('Origin',(0.,-1.84858989190502,0.));
#455890=CARTESIAN_POINT('',(-0.00189954774684422,4.65141010809498,-2.3697807159847));
#455891=CARTESIAN_POINT('',(-1.42212172806258E-5,4.84858989190502,-2.37515968171377));
#455892=CARTESIAN_POINT('',(-1.14631214242372E-14,-1.84858989190502,-2.37175));
#455893=CARTESIAN_POINT('',(-1.93106208855764,5.,1.37702479013102));
#455894=CARTESIAN_POINT('Ctrl Pts',(-0.00189954774684462,4.65141010809498,
-2.3697807159847));
#455895=CARTESIAN_POINT('Ctrl Pts',(-0.254987285068325,4.66836183412373,
-2.37158607092717));
#455896=CARTESIAN_POINT('Ctrl Pts',(-1.28591963123153,4.73756095222115,
-2.21873566508313));
#455897=CARTESIAN_POINT('Ctrl Pts',(-2.63119954910018,4.85375758285616,
-0.799366116563622));
#455898=CARTESIAN_POINT('Ctrl Pts',(-2.3348384767276,4.95300248746242,0.808908954735007));
#455899=CARTESIAN_POINT('Ctrl Pts',(-1.93307880200418,5.,1.37984525234445));
#455900=CARTESIAN_POINT('',(-1.93106208855765,5.,-1.37702479013102));
#455901=CARTESIAN_POINT('Origin',(0.,5.,0.));
#455902=CARTESIAN_POINT('Ctrl Pts',(-1.42212172806475E-5,4.84858989190502,
-2.37515968171377));
#455903=CARTESIAN_POINT('Ctrl Pts',(-0.747581930412603,4.89905992793668,
-2.37328899234637));
#455904=CARTESIAN_POINT('Ctrl Pts',(-1.49439019245277,4.94952996396834,
-1.98938888825773));
#455905=CARTESIAN_POINT('Ctrl Pts',(-1.93106208855765,5.,-1.37702479013102));
#455906=CARTESIAN_POINT('Origin',(0.,-1.84858989190502,0.));
#455907=CARTESIAN_POINT('',(0.0019133138563352,3.65141010809498,-2.37039078344507));
#455908=CARTESIAN_POINT('',(-0.00164128688419168,3.84858989190502,-2.36944791962108));
#455909=CARTESIAN_POINT('',(-1.14631214242372E-14,-1.84858989190502,-2.37175));
#455910=CARTESIAN_POINT('Ctrl Pts',(0.00191331385633514,3.65141010809498,
-2.37039078344507));
#455911=CARTESIAN_POINT('Ctrl Pts',(-0.547148555289758,3.68821081504498,
-2.36605148244037));
#455912=CARTESIAN_POINT('Ctrl Pts',(-1.88231140024366,3.77725891406365,
-1.90517491303348));
#455913=CARTESIAN_POINT('Ctrl Pts',(-2.77514400288091,3.91855440515103,
0.300097769845058));
#455914=CARTESIAN_POINT('Ctrl Pts',(-1.28464581100504,4.07529658135705,
2.47818845314823));
#455915=CARTESIAN_POINT('Ctrl Pts',(1.35445464728892,4.2320387575631,2.44071605927262));
#455916=CARTESIAN_POINT('Ctrl Pts',(2.78243358513013,4.38878093376914,0.221310557417421));
#455917=CARTESIAN_POINT('Ctrl Pts',(1.83787761908733,4.52857138394644,-1.93466620949292));
#455918=CARTESIAN_POINT('Ctrl Pts',(0.525061555809934,4.61611444205505,
-2.36602173562927));
#455919=CARTESIAN_POINT('Ctrl Pts',(-0.00189954774684462,4.65141010809498,
-2.3697807159847));
#455920=CARTESIAN_POINT('Ctrl Pts',(-0.00164128688419168,3.84858989190502,
-2.36944791962108));
#455921=CARTESIAN_POINT('Ctrl Pts',(-0.271541296495615,3.86666151678925,
-2.3712015367225));
#455922=CARTESIAN_POINT('Ctrl Pts',(-1.31965288321337,3.93698053374216,
-2.20510919750293));
#455923=CARTESIAN_POINT('Ctrl Pts',(-2.70764255999216,4.05954694276376,
-0.677933051861301));
#455924=CARTESIAN_POINT('Ctrl Pts',(-2.06245770113408,4.2162891189698,1.88123866225974));
#455925=CARTESIAN_POINT('Ctrl Pts',(0.427459215478939,4.37303129517583,
2.75839888164688));
#455926=CARTESIAN_POINT('Ctrl Pts',(2.53353286025567,4.52977347138188,1.16985680540038));
#455927=CARTESIAN_POINT('Ctrl Pts',(2.37788705609658,4.68651564758791,-1.46517155291796));
#455928=CARTESIAN_POINT('Ctrl Pts',(0.826561294082925,4.7927877877623,-2.36282686983047));
#455929=CARTESIAN_POINT('Ctrl Pts',(0.0263121713413973,4.846812535868,-2.37522556003093));
#455930=CARTESIAN_POINT('Ctrl Pts',(-1.42212172806475E-5,4.84858989190502,
-2.37515968171377));
#455931=CARTESIAN_POINT('Origin',(0.,-1.84858989190502,0.));
#455932=CARTESIAN_POINT('',(-0.0010854644346883,2.65141010809498,-2.37476211960784));
#455933=CARTESIAN_POINT('',(0.00198512898990283,2.84858989190502,-2.37083971328131));
#455934=CARTESIAN_POINT('',(-1.14631214242372E-14,-1.84858989190502,-2.37175));
#455935=CARTESIAN_POINT('Ctrl Pts',(-0.00108546443468895,2.65141010809498,
-2.37476211960784));
#455936=CARTESIAN_POINT('Ctrl Pts',(-0.0664545181996722,2.65581240389755,
-2.37513958979338));
#455937=CARTESIAN_POINT('Ctrl Pts',(-0.907265059639853,2.7124620917688,
-2.34333571530495));
#455938=CARTESIAN_POINT('Ctrl Pts',(-2.44564035685759,2.82135917170873,
-1.34552146026667));
#455939=CARTESIAN_POINT('Ctrl Pts',(-2.47349631950189,2.97810134791478,
1.29359897797797));
#455940=CARTESIAN_POINT('Ctrl Pts',(-0.29002949977508,3.13484352412081,
2.77623288044292));
#455941=CARTESIAN_POINT('Ctrl Pts',(2.15272817974667,3.29158570032686,1.77689322887057));
#455942=CARTESIAN_POINT('Ctrl Pts',(2.67092642591228,3.44832787653289,-0.811000349531056));
#455943=CARTESIAN_POINT('Ctrl Pts',(1.24026445200505,3.56826934578894,-2.23648619743872));
#455944=CARTESIAN_POINT('Ctrl Pts',(0.232375892058898,3.6359634229763,-2.37221215650581));
#455945=CARTESIAN_POINT('Ctrl Pts',(0.00191331385633514,3.65141010809498,
-2.37039078344507));
#455946=CARTESIAN_POINT('Ctrl Pts',(0.0019851289899029,2.84858989190502,
-2.37083971328131));
#455947=CARTESIAN_POINT('Ctrl Pts',(-0.563511833889923,2.8865104977105,
-2.36613048063736));
#455948=CARTESIAN_POINT('Ctrl Pts',(-1.91539516889925,2.97667849558466,
-1.88264567131773));
#455949=CARTESIAN_POINT('Ctrl Pts',(-2.76820658211993,3.11909388552752,
0.358615180585798));
#455950=CARTESIAN_POINT('Ctrl Pts',(-1.23202168904057,3.27583606173355,
2.50474086280712));
#455951=CARTESIAN_POINT('Ctrl Pts',(1.40561726678495,3.4325782379396,2.4116063446514));
#455952=CARTESIAN_POINT('Ctrl Pts',(2.78659025447549,3.58932041414563,0.162484526364377));
#455953=CARTESIAN_POINT('Ctrl Pts',(1.80439595705469,3.72799096546744,-1.95584969423954));
#455954=CARTESIAN_POINT('Ctrl Pts',(0.508774348159733,3.81441412472057,
-2.36613160411692));
#455955=CARTESIAN_POINT('Ctrl Pts',(-0.00164128688419168,3.84858989190502,
-2.36944791962108));
#455956=CARTESIAN_POINT('Origin',(0.,-1.84858989190502,0.));
#455957=CARTESIAN_POINT('',(-0.000430425503821624,1.65141010809498,-2.36815831308277));
#455958=CARTESIAN_POINT('',(-0.00131556418306894,1.84858989190502,-2.37442419787793));
#455959=CARTESIAN_POINT('',(-1.14631214242372E-14,-1.84858989190502,-2.37175));
#455960=CARTESIAN_POINT('Ctrl Pts',(-0.000430425503821948,1.65141010809498,
-2.36815831308277));
#455961=CARTESIAN_POINT('Ctrl Pts',(-0.363117743014602,1.6756613848188,
-2.36876395889577));
#455962=CARTESIAN_POINT('Ctrl Pts',(-1.50640329832999,1.7521600536113,-2.12141555137754));
#455963=CARTESIAN_POINT('Ctrl Pts',(-2.76820605062014,1.88090611447249,
-0.358615115250419));
#455964=CARTESIAN_POINT('Ctrl Pts',(-1.82960322615152,2.03764829067853,
2.10811294705418));
#455965=CARTESIAN_POINT('Ctrl Pts',(0.744683162267116,2.19439046688457,
2.69017343400533));
#455966=CARTESIAN_POINT('Ctrl Pts',(2.65321484974249,2.35113264309061,0.867198546770537));
#455967=CARTESIAN_POINT('Ctrl Pts',(2.2027709898381,2.50347252349408,-1.65808273322866));
#455968=CARTESIAN_POINT('Ctrl Pts',(0.70935945123483,2.60356501182887,-2.37065969256184));
#455969=CARTESIAN_POINT('Ctrl Pts',(-0.00108546443468895,2.65141010809498,
-2.37476211960784));
#455970=CARTESIAN_POINT('Ctrl Pts',(-0.00131556418306908,1.84858989190502,
-2.37442419787793));
#455971=CARTESIAN_POINT('Ctrl Pts',(-0.0833447701680231,1.85411208656308,
-2.3749769878955));
#455972=CARTESIAN_POINT('Ctrl Pts',(-0.940926068943489,1.91188167328981,
-2.33425678779921));
#455973=CARTESIAN_POINT('Ctrl Pts',(-2.4734967778431,2.02189865208523,-1.29359921657332));
#455974=CARTESIAN_POINT('Ctrl Pts',(-2.44564080514743,2.17864082829127,
1.34552170813359));
#455975=CARTESIAN_POINT('Ctrl Pts',(-0.231363468903584,2.33538300449731,
2.78173658695524));
#455976=CARTESIAN_POINT('Ctrl Pts',(2.18975452958847,2.49212518070335,1.73105826447513));
#455977=CARTESIAN_POINT('Ctrl Pts',(2.65321534120238,2.64886735690939,-0.867198706368743));
#455978=CARTESIAN_POINT('Ctrl Pts',(1.20641409926552,2.76768892730995,-2.24914186907922));
#455979=CARTESIAN_POINT('Ctrl Pts',(0.215635569102197,2.83426310564182,
-2.37261890873773));
#455980=CARTESIAN_POINT('Ctrl Pts',(0.0019851289899029,2.84858989190502,
-2.37083971328131));
#455981=CARTESIAN_POINT('Origin',(0.,-1.84858989190502,0.));
#455982=CARTESIAN_POINT('',(0.00189242379211233,0.651410108094979,-2.37343051434144));
#455983=CARTESIAN_POINT('',(-0.000162827624894668,0.848589891905021,-2.36808927594338));
#455984=CARTESIAN_POINT('',(-1.14631214242372E-14,-1.84858989190502,-2.37175));
#455985=CARTESIAN_POINT('Ctrl Pts',(0.00189242379211238,0.651410108094979,
-2.37343051434144));
#455986=CARTESIAN_POINT('Ctrl Pts',(-0.653878033681435,0.695510365740054,
-2.36800951817008));
#455987=CARTESIAN_POINT('Ctrl Pts',(-2.09599365201939,0.79185801545381,
-1.74821763141818));
#455988=CARTESIAN_POINT('Ctrl Pts',(-2.7076414341639,0.940453057236244,
0.677932800861099));
#455989=CARTESIAN_POINT('Ctrl Pts',(-0.932633404653946,1.09719523344229,
2.63093846489754));
#455990=CARTESIAN_POINT('Ctrl Pts',(1.67639574619592,1.25393740964833,2.23191177495579));
#455991=CARTESIAN_POINT('Ctrl Pts',(2.78658961819278,1.41067958585437,-0.162484485327371));
#455992=CARTESIAN_POINT('Ctrl Pts',(1.61928227105817,1.54317048533659,-2.06362001410675));
#455993=CARTESIAN_POINT('Ctrl Pts',(0.41826241655896,1.62341399275012,-2.36745914453045));
#455994=CARTESIAN_POINT('Ctrl Pts',(-0.000430425503821948,1.65141010809498,
-2.36815831308277));
#455995=CARTESIAN_POINT('Ctrl Pts',(-0.00016282762489446,0.848589891905021,
-2.36808927594338));
#455996=CARTESIAN_POINT('Ctrl Pts',(-0.3796310646964,0.873961067484328,
-2.36834769891036));
#455997=CARTESIAN_POINT('Ctrl Pts',(-1.54021819528391,0.951579635132315,
-2.10471668851161));
#455998=CARTESIAN_POINT('Ctrl Pts',(-2.77514463720035,1.08144559484898,
-0.300097834486946));
#455999=CARTESIAN_POINT('Ctrl Pts',(-1.78470554216421,1.23818777105502,
2.14625981419194));
#456000=CARTESIAN_POINT('Ctrl Pts',(0.801305687705963,1.39492994726106,
2.67385740587119));
#456001=CARTESIAN_POINT('Ctrl Pts',(2.67092693931563,1.5516721234671,0.811000501773433));
#456002=CARTESIAN_POINT('Ctrl Pts',(2.17098524681304,1.70289210501509,-1.68571927954979));
#456003=CARTESIAN_POINT('Ctrl Pts',(0.692761896033403,1.8018646944944,-2.36974685050122));
#456004=CARTESIAN_POINT('Ctrl Pts',(-0.00131556418306908,1.84858989190502,
-2.37442419787793));
#456005=CARTESIAN_POINT('Ctrl Pts',(2.13201587949045,-0.329233991005384,
-1.03908919352506));
#456006=CARTESIAN_POINT('Ctrl Pts',(1.79090363105035,-0.276986598936704,
-1.73898746491002));
#456007=CARTESIAN_POINT('Ctrl Pts',(0.372188007793122,-0.172491814799343,
-2.76564966890019));
#456008=CARTESIAN_POINT('Ctrl Pts',(-2.10316535941187,-0.0157496385933029,
-1.8378710515163));
#456009=CARTESIAN_POINT('Ctrl Pts',(-2.69198404294186,0.140992537612738,
0.735238472662612));
#456010=CARTESIAN_POINT('Ctrl Pts',(-0.877278354639368,0.297734713818778,
2.64988083876425));
#456011=CARTESIAN_POINT('Ctrl Pts',(1.72333502783425,0.454476890024819,
2.1961118038906));
#456012=CARTESIAN_POINT('Ctrl Pts',(2.78243473695495,0.61121906623086,-0.221310618979959));
#456013=CARTESIAN_POINT('Ctrl Pts',(1.35445452184974,0.7679612424369,-2.44071651245848));
#456014=CARTESIAN_POINT('Ctrl Pts',(-1.2846458307181,0.924703418642942,
-2.47818889868423));
#456015=CARTESIAN_POINT('Ctrl Pts',(-2.77514463720035,1.08144559484898,
-0.300097834486946));
#456016=CARTESIAN_POINT('Ctrl Pts',(-1.78470554216421,1.23818777105502,
2.14625981419194));
#456017=CARTESIAN_POINT('Ctrl Pts',(0.801305687705963,1.39492994726106,
2.67385740587119));
#456018=CARTESIAN_POINT('Ctrl Pts',(2.67092693931563,1.5516721234671,0.811000501773433));
#456019=CARTESIAN_POINT('Ctrl Pts',(2.15272856330194,1.70841429967315,-1.77689355756481));
#456020=CARTESIAN_POINT('Ctrl Pts',(-0.290029546396374,1.86515647587919,
-2.77623338981819));
#456021=CARTESIAN_POINT('Ctrl Pts',(-2.4734967778431,2.02189865208523,-1.29359921657332));
#456022=CARTESIAN_POINT('Ctrl Pts',(-2.44564080514743,2.17864082829127,
1.34552170813359));
#456023=CARTESIAN_POINT('Ctrl Pts',(-0.231363468903584,2.33538300449731,
2.78173658695524));
#456024=CARTESIAN_POINT('Ctrl Pts',(2.18975452958847,2.49212518070335,1.73105826447513));
#456025=CARTESIAN_POINT('Ctrl Pts',(2.65321534120238,2.64886735690939,-0.867198706368743));
#456026=CARTESIAN_POINT('Ctrl Pts',(0.744683292397524,2.80560953311543,
-2.69017392867975));
#456027=CARTESIAN_POINT('Ctrl Pts',(-1.82960355013577,2.96235170932147,
-2.10811333459611));
#456028=CARTESIAN_POINT('Ctrl Pts',(-2.76820658211993,3.11909388552752,
0.358615180585798));
#456029=CARTESIAN_POINT('Ctrl Pts',(-1.23202168904057,3.27583606173355,
2.50474086280712));
#456030=CARTESIAN_POINT('Ctrl Pts',(1.40561726678495,3.4325782379396,2.4116063446514));
#456031=CARTESIAN_POINT('Ctrl Pts',(2.78659025447549,3.58932041414563,0.162484526364377));
#456032=CARTESIAN_POINT('Ctrl Pts',(1.67639583924145,3.74606259035167,-2.2319122111134));
#456033=CARTESIAN_POINT('Ctrl Pts',(-0.932633206071211,3.90280476655772,
-2.63093889113374));
#456034=CARTESIAN_POINT('Ctrl Pts',(-2.70764255999216,4.05954694276376,
-0.677933051861301));
#456035=CARTESIAN_POINT('Ctrl Pts',(-2.06245770113408,4.2162891189698,1.88123866225974));
#456036=CARTESIAN_POINT('Ctrl Pts',(0.427459215478939,4.37303129517583,
2.75839888164688));
#456037=CARTESIAN_POINT('Ctrl Pts',(2.53353286025567,4.52977347138188,1.16985680540038));
#456038=CARTESIAN_POINT('Ctrl Pts',(2.37788705609658,4.68651564758791,-1.46517155291796));
#456039=CARTESIAN_POINT('Ctrl Pts',(0.0898163016776116,4.84325782379396,
-2.7891351771088));
#456040=CARTESIAN_POINT('Ctrl Pts',(-1.47901232685639,4.94775260793132,
-2.01095394174764));
#456041=CARTESIAN_POINT('Ctrl Pts',(-1.93106208855765,5.,-1.37702479013102));
#456042=CARTESIAN_POINT('Ctrl Pts',(2.30288577939269,-0.219489327336923,
-1.12236674703445));
#456043=CARTESIAN_POINT('Ctrl Pts',(1.93443517184041,-0.167241935268243,
-1.87835819705084));
#456044=CARTESIAN_POINT('Ctrl Pts',(0.402016926164794,-0.0627471511308819,
-2.98730199646287));
#456045=CARTESIAN_POINT('Ctrl Pts',(-2.2717230413211,0.0939950250751584,
-1.98516678492372));
#456046=CARTESIAN_POINT('Ctrl Pts',(-2.90773245662903,0.250737201281199,
0.794163983225957));
#456047=CARTESIAN_POINT('Ctrl Pts',(-0.947587617382505,0.40747937748724,
2.86225490127861));
#456048=CARTESIAN_POINT('Ctrl Pts',(1.86145129917011,0.564221553693281,
2.37211865623853));
#456049=CARTESIAN_POINT('Ctrl Pts',(3.00543229975999,0.720963729899321,
-0.239047505311898));
#456050=CARTESIAN_POINT('Ctrl Pts',(1.46300695375092,0.877705906105364,
-2.63632715034604));
#456051=CARTESIAN_POINT('Ctrl Pts',(-1.38760346185783,1.0344480823114,-2.67680275195357));
#456052=CARTESIAN_POINT('Ctrl Pts',(-2.99755793671386,1.19119025851744,
-0.324149103257007));
#456053=CARTESIAN_POINT('Ctrl Pts',(-1.92774033861116,1.34793243472348,
2.3182712908151));
#456054=CARTESIAN_POINT('Ctrl Pts',(0.865526139329494,1.50467461092953,
2.88815306458986));
#456055=CARTESIAN_POINT('Ctrl Pts',(2.884987736497,1.66141678713557,0.875997941938753));
#456056=CARTESIAN_POINT('Ctrl Pts',(2.32525847626676,1.81815896334161,-1.91930226438486));
#456057=CARTESIAN_POINT('Ctrl Pts',(-0.313273894638884,1.97490113954765,
-2.9987339471484));
#456058=CARTESIAN_POINT('Ctrl Pts',(-2.6717345822161,2.13164331575369,-1.39727441466909));
#456059=CARTESIAN_POINT('Ctrl Pts',(-2.64164609928823,2.28838549195973,
1.45335822182786));
#456060=CARTESIAN_POINT('Ctrl Pts',(-0.2499060384749,2.44512766816577,3.00467819669646));
#456061=CARTESIAN_POINT('Ctrl Pts',(2.36525187971641,2.60186984437181,1.8697935127541));
#456062=CARTESIAN_POINT('Ctrl Pts',(2.86585664661268,2.75861202057785,-0.936700138125429));
#456063=CARTESIAN_POINT('Ctrl Pts',(0.804365755767006,2.91535419678389,
-2.90577727119472));
#456064=CARTESIAN_POINT('Ctrl Pts',(-1.97623668663343,3.07209637298993,
-2.27706757078646));
#456065=CARTESIAN_POINT('Ctrl Pts',(-2.99006383287765,3.22883854919597,
0.387356307985263));
#456066=CARTESIAN_POINT('Ctrl Pts',(-1.33076177100191,3.38558072540201,
2.70548271685522));
#456067=CARTESIAN_POINT('Ctrl Pts',(1.51827012457408,3.54232290160805,2.60488395514119));
#456068=CARTESIAN_POINT('Ctrl Pts',(3.00992086023279,3.6990650778141,0.175506809651583));
#456069=CARTESIAN_POINT('Ctrl Pts',(1.81075018059663,3.85580725402013,-2.41078827848804));
#456070=CARTESIAN_POINT('Ctrl Pts',(-1.00737887006926,4.01254943022618,
-2.84179485581088));
#456071=CARTESIAN_POINT('Ctrl Pts',(-2.92464592176238,4.16929160643222,
-0.732265833256742));
#456072=CARTESIAN_POINT('Ctrl Pts',(-2.22775287756101,4.32603378263826,
2.03201008240009));
#456073=CARTESIAN_POINT('Ctrl Pts',(0.461717831497611,4.48277595884429,
2.97947009660899));
#456074=CARTESIAN_POINT('Ctrl Pts',(2.73658224201468,4.63951813505034,1.26361469771331));
#456075=CARTESIAN_POINT('Ctrl Pts',(2.56846224231478,4.79626031125638,-1.58259737464615));
#456076=CARTESIAN_POINT('Ctrl Pts',(0.0970146075743366,4.95300248746242,
-3.01266974507848));
#456077=CARTESIAN_POINT('Ctrl Pts',(-1.5975474140831,5.05749727159978,-2.17212136176543));
#456078=CARTESIAN_POINT('Ctrl Pts',(-2.08582659521588,5.10974466366846,
-1.48738611075535));
#456079=CARTESIAN_POINT('Ctrl Pts',(2.47375567929493,-0.109744663668462,
-1.20564430054383));
#456080=CARTESIAN_POINT('Ctrl Pts',(2.07796671263047,-0.0574972715997812,
-2.01772892919166));
#456081=CARTESIAN_POINT('Ctrl Pts',(0.431845844536463,0.0469975125375793,
-3.20895432402555));
#456082=CARTESIAN_POINT('Ctrl Pts',(-2.44028072323032,0.20373968874362,
-2.13246251833114));
#456083=CARTESIAN_POINT('Ctrl Pts',(-3.1234808703162,0.360481864949661,
0.853089493789302));
#456084=CARTESIAN_POINT('Ctrl Pts',(-1.01789688012564,0.517224041155701,
3.07462896379297));
#456085=CARTESIAN_POINT('Ctrl Pts',(1.99956757050596,0.673966217361742,
2.54812550858646));
#456086=CARTESIAN_POINT('Ctrl Pts',(3.22842986256503,0.830708393567783,
-0.256784391643832));
#456087=CARTESIAN_POINT('Ctrl Pts',(1.57155938565209,0.987450569773824,
-2.8319377882336));
#456088=CARTESIAN_POINT('Ctrl Pts',(-1.49056109299756,1.14419274597986,
-2.87541660522291));
#456089=CARTESIAN_POINT('Ctrl Pts',(-3.21997123622737,1.30093492218591,
-0.348200372027069));
#456090=CARTESIAN_POINT('Ctrl Pts',(-2.07077513505811,1.45767709839195,
2.49028276743826));
#456091=CARTESIAN_POINT('Ctrl Pts',(0.929746590953023,1.61441927459799,
3.10244872330854));
#456092=CARTESIAN_POINT('Ctrl Pts',(3.09904853367837,1.77116145080403,0.940995382104076));
#456093=CARTESIAN_POINT('Ctrl Pts',(2.49778838923158,1.92790362701007,-2.0617109712049));
#456094=CARTESIAN_POINT('Ctrl Pts',(-0.336518242881397,2.08464580321611,
-3.22123450447862));
#456095=CARTESIAN_POINT('Ctrl Pts',(-2.8699723865891,2.24138797942214,-1.50094961276486));
#456096=CARTESIAN_POINT('Ctrl Pts',(-2.83765139342903,2.3981301556282,1.56119473552213));
#456097=CARTESIAN_POINT('Ctrl Pts',(-0.268448608046208,2.55487233183423,
3.22761980643768));
#456098=CARTESIAN_POINT('Ctrl Pts',(2.54074922984435,2.71161450804027,2.00852876103307));
#456099=CARTESIAN_POINT('Ctrl Pts',(3.07849795202298,2.86835668424631,-1.00620156988212));
#456100=CARTESIAN_POINT('Ctrl Pts',(0.864048219136484,3.02509886045235,
-3.12138061370969));
#456101=CARTESIAN_POINT('Ctrl Pts',(-2.12286982313108,3.18184103665839,
-2.44602180697682));
#456102=CARTESIAN_POINT('Ctrl Pts',(-3.21192108363538,3.33858321286443,
0.416097435384728));
#456103=CARTESIAN_POINT('Ctrl Pts',(-1.42950185296324,3.49532538907048,
2.90622457090332));
#456104=CARTESIAN_POINT('Ctrl Pts',(1.63092298236321,3.65206756527651,2.79816156563098));
#456105=CARTESIAN_POINT('Ctrl Pts',(3.23325146599009,3.80880974148256,0.188529092938788));
#456106=CARTESIAN_POINT('Ctrl Pts',(1.94510452195181,3.96555191768859,-2.58966434586268));
#456107=CARTESIAN_POINT('Ctrl Pts',(-1.08212453406731,4.12229409389464,
-3.05265082048802));
#456108=CARTESIAN_POINT('Ctrl Pts',(-3.14164928353259,4.27903627010068,
-0.786598614652181));
#456109=CARTESIAN_POINT('Ctrl Pts',(-2.39304805398794,4.43577844630672,
2.18278150254044));
#456110=CARTESIAN_POINT('Ctrl Pts',(0.495976447516285,4.59252062251276,
3.2005413115711));
#456111=CARTESIAN_POINT('Ctrl Pts',(2.93963162377369,4.7492627987188,1.35737259002624));
#456112=CARTESIAN_POINT('Ctrl Pts',(2.75903742853299,4.90600497492484,-1.70002319637433));
#456113=CARTESIAN_POINT('Ctrl Pts',(0.10421291347106,5.06274715113088,-3.23620431304816));
#456114=CARTESIAN_POINT('Ctrl Pts',(-1.71608250130981,5.16724193526824,
-2.33328878178322));
#456115=CARTESIAN_POINT('Ctrl Pts',(-2.24059110187411,5.21948932733692,
-1.59774743137967));
#456116=CARTESIAN_POINT('Ctrl Pts',(2.64462557919718,-2.77555756156289E-16,
-1.28892185405322));
#456117=CARTESIAN_POINT('Ctrl Pts',(2.22149825342052,0.05224739206868,-2.15709966133247));
#456118=CARTESIAN_POINT('Ctrl Pts',(0.461674762908137,0.156742176206041,
-3.43060665158822));
#456119=CARTESIAN_POINT('Ctrl Pts',(-2.60883840513955,0.313484352412081,
-2.27975825173857));
#456120=CARTESIAN_POINT('Ctrl Pts',(-3.33922928400336,0.470226528618122,
0.91201500435265));
#456121=CARTESIAN_POINT('Ctrl Pts',(-1.08820614286878,0.626968704824163,
3.28700302630733));
#456122=CARTESIAN_POINT('Ctrl Pts',(2.13768384184183,0.783710881030202,
2.72413236093439));
#456123=CARTESIAN_POINT('Ctrl Pts',(3.45142742537007,0.940453057236245,
-0.27452127797577));
#456124=CARTESIAN_POINT('Ctrl Pts',(1.68011181755326,1.09719523344228,-3.02754842612115));
#456125=CARTESIAN_POINT('Ctrl Pts',(-1.5935187241373,1.25393740964832,-3.07403045849226));
#456126=CARTESIAN_POINT('Ctrl Pts',(-3.44238453574088,1.41067958585437,
-0.372251640797132));
#456127=CARTESIAN_POINT('Ctrl Pts',(-2.21380993150506,1.5674217620604,2.66229424406142));
#456128=CARTESIAN_POINT('Ctrl Pts',(0.993967042576552,1.72416393826645,
3.31674438202721));
#456129=CARTESIAN_POINT('Ctrl Pts',(3.31310933085974,1.88090611447249,1.0059928222694));
#456130=CARTESIAN_POINT('Ctrl Pts',(2.67031830219639,2.03764829067853,-2.20411967802495));
#456131=CARTESIAN_POINT('Ctrl Pts',(-0.359762591123905,2.19439046688457,
-3.44373506180883));
#456132=CARTESIAN_POINT('Ctrl Pts',(-3.06821019096211,2.35113264309061,
-1.60462481086063));
#456133=CARTESIAN_POINT('Ctrl Pts',(-3.03365668756983,2.50787481929665,
1.6690312492164));
#456134=CARTESIAN_POINT('Ctrl Pts',(-0.286991177617524,2.6646169955027,
3.45056141617891));
#456135=CARTESIAN_POINT('Ctrl Pts',(2.71624657997229,2.82135917170873,2.14726400931204));
#456136=CARTESIAN_POINT('Ctrl Pts',(3.29113925743328,2.97810134791478,-1.0757030016388));
#456137=CARTESIAN_POINT('Ctrl Pts',(0.923730682505967,3.13484352412081,
-3.33698395622466));
#456138=CARTESIAN_POINT('Ctrl Pts',(-2.26950295962873,3.29158570032686,
-2.61497604316717));
#456139=CARTESIAN_POINT('Ctrl Pts',(-3.43377833439311,3.4483278765329,0.444838562784192));
#456140=CARTESIAN_POINT('Ctrl Pts',(-1.52824193492458,3.60507005273893,
3.10696642495143));
#456141=CARTESIAN_POINT('Ctrl Pts',(1.74357584015234,3.76181222894498,2.99143917612077));
#456142=CARTESIAN_POINT('Ctrl Pts',(3.4565820717474,3.91855440515102,0.201551376225996));
#456143=CARTESIAN_POINT('Ctrl Pts',(2.07945886330698,4.07529658135705,-2.76854041323733));
#456144=CARTESIAN_POINT('Ctrl Pts',(-1.15687019806535,4.2320387575631,-3.26350678516516));
#456145=CARTESIAN_POINT('Ctrl Pts',(-3.35865264530281,4.38878093376914,
-0.840931396047624));
#456146=CARTESIAN_POINT('Ctrl Pts',(-2.55834323041487,4.54552310997518,
2.33355292268079));
#456147=CARTESIAN_POINT('Ctrl Pts',(0.530235063534957,4.70226528618122,
3.42161252653321));
#456148=CARTESIAN_POINT('Ctrl Pts',(3.1426810055327,4.85900746238726,1.45113048233917));
#456149=CARTESIAN_POINT('Ctrl Pts',(2.94961261475119,5.0157496385933,-1.81744901810252));
#456150=CARTESIAN_POINT('Ctrl Pts',(0.111411219367783,5.17249181479934,
-3.45973888101785));
#456151=CARTESIAN_POINT('Ctrl Pts',(-1.83461758853652,5.2769865989367,-2.49445620180102));
#456152=CARTESIAN_POINT('Ctrl Pts',(-2.39535560853235,5.32923399100538,
-1.70810875200399));
#456153=CARTESIAN_POINT('',(2.64462557919717,5.,-1.28892185405324));
#456154=CARTESIAN_POINT('Ctrl Pts',(2.64766952698147,5.,-1.2919603520133));
#456155=CARTESIAN_POINT('Ctrl Pts',(2.59777169898683,5.,-1.37498714432249));
#456156=CARTESIAN_POINT('Ctrl Pts',(2.54371038927642,5.,-1.45514089331332));
#456157=CARTESIAN_POINT('Ctrl Pts',(2.48549510771317,5.,-1.53206201799603));
#456158=CARTESIAN_POINT('Ctrl Pts',(2.42718170236622,5.,-1.60911279578009));
#456159=CARTESIAN_POINT('Ctrl Pts',(2.36469961903881,5.,-1.68292056059732));
#456160=CARTESIAN_POINT('Ctrl Pts',(2.2984276527278,5.,-1.75333415410535));
#456161=CARTESIAN_POINT('Ctrl Pts',(2.22837518703592,5.,-1.82776450705904));
#456162=CARTESIAN_POINT('Ctrl Pts',(2.15408724664126,5.,-1.89840328930852));
#456163=CARTESIAN_POINT('Ctrl Pts',(2.07598025051918,5.,-1.965018936113));
#456164=CARTESIAN_POINT('Ctrl Pts',(2.04180843971577,5.,-1.99416328158996));
#456165=CARTESIAN_POINT('Ctrl Pts',(2.006905334995,5.,-2.02253683217268));
#456166=CARTESIAN_POINT('Ctrl Pts',(1.97130480013543,5.,-2.05011658752475));
#456167=CARTESIAN_POINT('Ctrl Pts',(1.94660081204988,5.,-2.06925478166446));
#456168=CARTESIAN_POINT('Ctrl Pts',(1.92156098161269,5.,-2.08801069507471));
#456169=CARTESIAN_POINT('Ctrl Pts',(1.89619655797919,5.,-2.10637598129296));
#456170=CARTESIAN_POINT('Ctrl Pts',(1.88438047127152,5.,-2.11493150053131));
#456171=CARTESIAN_POINT('Ctrl Pts',(1.87250080990167,5.,-2.12339724242785));
#456172=CARTESIAN_POINT('Ctrl Pts',(1.8605620114611,5.,-2.13177054329346));
#456173=CARTESIAN_POINT('Ctrl Pts',(1.78200362920114,5.,-2.18686762642564));
#456174=CARTESIAN_POINT('Ctrl Pts',(1.70084366480229,5.,-2.23799730804012));
#456175=CARTESIAN_POINT('Ctrl Pts',(1.61744916104773,5.,-2.28501302782822));
#456176=CARTESIAN_POINT('Ctrl Pts',(1.53432547022518,5.,-2.33187607010938));
#456177=CARTESIAN_POINT('Ctrl Pts',(1.44898075932165,5.,-2.37465210593129));
#456178=CARTESIAN_POINT('Ctrl Pts',(1.36176167588437,5.,-2.41314743430364));
#456179=CARTESIAN_POINT('Ctrl Pts',(1.27604812534558,5.,-2.45097827526087));
#456180=CARTESIAN_POINT('Ctrl Pts',(1.18852347245503,5.,-2.48467505469784));
#456181=CARTESIAN_POINT('Ctrl Pts',(1.09951413378954,5.,-2.51400404744347));
#456182=CARTESIAN_POINT('Ctrl Pts',(1.05865424614969,5.,-2.5274675712281));
#456183=CARTESIAN_POINT('Ctrl Pts',(1.01748153675728,5.,-2.54000996680563));
#456184=CARTESIAN_POINT('Ctrl Pts',(0.976028153801408,5.,-2.55160488811041));
#456185=CARTESIAN_POINT('Ctrl Pts',(0.957566358606986,5.,-2.55676883486603));
#456186=CARTESIAN_POINT('Ctrl Pts',(0.939048899883842,5.,-2.56174481989958));
#456187=CARTESIAN_POINT('Ctrl Pts',(0.920478659872387,5.,-2.56653035938024));
#456188=CARTESIAN_POINT('Ctrl Pts',(0.907359430777782,5.,-2.5699111766852));
#456189=CARTESIAN_POINT('Ctrl Pts',(0.894223325226895,5.,-2.57319450150697));
#456190=CARTESIAN_POINT('Ctrl Pts',(0.881071607747158,5.,-2.57637981427696));
#456191=CARTESIAN_POINT('Ctrl Pts',(0.791886436427642,5.,-2.59798023760843));
#456192=CARTESIAN_POINT('Ctrl Pts',(0.701979962263147,5.,-2.61507864060924));
#456193=CARTESIAN_POINT('Ctrl Pts',(0.611667974021129,5.,-2.62750345202927));
#456194=CARTESIAN_POINT('Ctrl Pts',(0.523982886910535,5.,-2.6395668634645));
#456195=CARTESIAN_POINT('Ctrl Pts',(0.435914782332347,5.,-2.6472245845699));
#456196=CARTESIAN_POINT('Ctrl Pts',(0.347756020174879,5.,-2.65027173618512));
#456197=CARTESIAN_POINT('Ctrl Pts',(0.261159272931329,5.,-2.65326489774705));
#456198=CARTESIAN_POINT('Ctrl Pts',(0.174474421690037,5.,-2.65180947160144));
#456199=CARTESIAN_POINT('Ctrl Pts',(0.087991872332091,5.,-2.645664129397));
#456200=CARTESIAN_POINT('Ctrl Pts',(0.0366551246938374,5.,-2.64201620407285));
#456201=CARTESIAN_POINT('Ctrl Pts',(-0.0146100375789589,5.,-2.63671460852521));
#456202=CARTESIAN_POINT('Ctrl Pts',(-0.0657395497789789,5.,-2.62978719346761));
#456203=CARTESIAN_POINT('Ctrl Pts',(-0.0799569026170698,5.,-2.6278609184086));
#456204=CARTESIAN_POINT('Ctrl Pts',(-0.0941655555404146,5.,-2.62580863159305));
#456205=CARTESIAN_POINT('Ctrl Pts',(-0.108358376628224,5.,-2.62363175914501));
#456206=CARTESIAN_POINT('Ctrl Pts',(-0.195234128720159,5.,-2.61030689371046));
#456207=CARTESIAN_POINT('Ctrl Pts',(-0.281231397385426,5.,-2.59236346059264));
#456208=CARTESIAN_POINT('Ctrl Pts',(-0.366064031431315,5.,-2.57003255344105));
#456209=CARTESIAN_POINT('Ctrl Pts',(-0.452588039204867,5.,-2.54725641775098));
#456210=CARTESIAN_POINT('Ctrl Pts',(-0.537901385141664,5.,-2.51991561409353));
#456211=CARTESIAN_POINT('Ctrl Pts',(-0.621678841171493,5.,-2.48820642097155));
#456212=CARTESIAN_POINT('Ctrl Pts',(-0.704710490888595,5.,-2.45677951042919));
#456213=CARTESIAN_POINT('Ctrl Pts',(-0.786234206302495,5.,-2.42106095415721));
#456214=CARTESIAN_POINT('Ctrl Pts',(-0.865900432570674,5.,-2.38120349844864));
#456215=CARTESIAN_POINT('Ctrl Pts',(-0.901637362928322,5.,-2.36332411359997));
#456216=CARTESIAN_POINT('Ctrl Pts',(-0.937000006729313,5.,-2.34461141659527));
#456217=CARTESIAN_POINT('Ctrl Pts',(-0.971954039217656,5.,-2.32507720525684));
#456218=CARTESIAN_POINT('Ctrl Pts',(-0.992269863313026,5.,-2.31372361961473));
#456219=CARTESIAN_POINT('Ctrl Pts',(-1.01244761935627,5.,-2.30209249607874));
#456220=CARTESIAN_POINT('Ctrl Pts',(-1.03248026178061,5.,-2.29018599166716));
#456221=CARTESIAN_POINT('Ctrl Pts',(-1.04555625392411,5.,-2.28241420825265));
#456222=CARTESIAN_POINT('Ctrl Pts',(-1.05856245336876,5.,-2.27452980761246));
#456223=CARTESIAN_POINT('Ctrl Pts',(-1.07149500085763,5.,-2.26653512611973));
#456224=CARTESIAN_POINT('Ctrl Pts',(-1.14590971351802,5.,-2.22053321299281));
#456225=CARTESIAN_POINT('Ctrl Pts',(-1.21791340134486,5.,-2.17086827794226));
#456226=CARTESIAN_POINT('Ctrl Pts',(-1.28718056809639,5.,-2.1177080547548));
#456227=CARTESIAN_POINT('Ctrl Pts',(-1.35260286286025,5.,-2.06749864163476));
#456228=CARTESIAN_POINT('Ctrl Pts',(-1.41558423704355,5.,-2.01417045251016));
#456229=CARTESIAN_POINT('Ctrl Pts',(-1.47581393671382,5.,-1.95784078111152));
#456230=CARTESIAN_POINT('Ctrl Pts',(-1.49258058151295,5.,-1.94215981977247));
#456231=CARTESIAN_POINT('Ctrl Pts',(-1.50913374759254,5.,-1.92624614509165));
#456232=CARTESIAN_POINT('Ctrl Pts',(-1.52546615283854,5.,-1.91010204310153));
#456233=CARTESIAN_POINT('Ctrl Pts',(-1.54179078985554,5.,-1.89396561977719));
#456234=CARTESIAN_POINT('Ctrl Pts',(-1.55789860538532,5.,-1.87759488117163));
#456235=CARTESIAN_POINT('Ctrl Pts',(-1.57376018959548,5.,-1.86101550415345));
#456236=CARTESIAN_POINT('Ctrl Pts',(-1.63176973842762,5.,-1.80038081798342));
#456237=CARTESIAN_POINT('Ctrl Pts',(-1.68654047451408,5.,-1.73690977802179));
#456238=CARTESIAN_POINT('Ctrl Pts',(-1.73775463425817,5.,-1.67073898254984));
#456239=CARTESIAN_POINT('Ctrl Pts',(-1.78752683631336,5.,-1.60643125556886));
#456240=CARTESIAN_POINT('Ctrl Pts',(-1.83394024106878,5.,-1.53957306420248));
#456241=CARTESIAN_POINT('Ctrl Pts',(-1.87665739561666,5.,-1.47027246234511));
#456242=CARTESIAN_POINT('Ctrl Pts',(-1.89552476650306,5.,-1.43966367831601));
#456243=CARTESIAN_POINT('Ctrl Pts',(-1.91367042541382,5.,-1.40857824435308));
#456244=CARTESIAN_POINT('Ctrl Pts',(-1.93106208855765,5.,-1.37702479013102));
#456245=CARTESIAN_POINT('Ctrl Pts',(-0.00203590851197863,4.17782388291041,
-2.93914442058615));
#456246=CARTESIAN_POINT('Ctrl Pts',(-0.336829132197776,4.19589550779464,
-2.9413196673501));
#456247=CARTESIAN_POINT('Ctrl Pts',(-0.670951610256496,4.21396713267887,
-2.8883718851961));
#456248=CARTESIAN_POINT('Ctrl Pts',(-0.984445762376185,4.2320387575631,
-2.77724982499094));
#456249=CARTESIAN_POINT('Ctrl Pts',(-1.89079768047782,4.28428614963178,
-2.45598165545933));
#456250=CARTESIAN_POINT('Ctrl Pts',(-2.62472516289032,4.33653354170046,
-1.64845652575348));
#456251=CARTESIAN_POINT('Ctrl Pts',(-2.85830400161524,4.38878093376914,
-0.715613241112485));
#456252=CARTESIAN_POINT('Ctrl Pts',(-3.09188284034016,4.44102832583782,
0.21723004352851));
#456253=CARTESIAN_POINT('Ctrl Pts',(-2.82511303537752,4.4932757179065,1.27539148310465));
#456254=CARTESIAN_POINT('Ctrl Pts',(-2.17696508390455,4.54552310997518,
1.98581547020146));
#456255=CARTESIAN_POINT('Ctrl Pts',(-1.52881713243159,4.59777050204386,
2.69623945729826));
#456256=CARTESIAN_POINT('Ctrl Pts',(-0.499291034448317,4.65001789411254,
3.05892599191573));
#456257=CARTESIAN_POINT('Ctrl Pts',(0.450879671542943,4.70226528618122,
2.91185558519213));
#456258=CARTESIAN_POINT('Ctrl Pts',(1.4010503775342,4.7545126782499,2.76478517846853));
#456259=CARTESIAN_POINT('Ctrl Pts',(2.27186569153346,4.80676007031858,2.10795783040384));
#456260=CARTESIAN_POINT('Ctrl Pts',(2.67509528340283,4.85900746238726,1.23478090629788));
#456261=CARTESIAN_POINT('Ctrl Pts',(3.03780789065589,4.90600497492484,0.449341828606679));
#456262=CARTESIAN_POINT('Ctrl Pts',(3.02218094071591,4.95300248746242,-0.511153070775355));
#456263=CARTESIAN_POINT('Ctrl Pts',(2.64766952698147,5.,-1.2919603520133));
#456264=CARTESIAN_POINT('',(-1.933077639016,-4.14165229889463E-16,-1.37984607144989));
#456265=CARTESIAN_POINT('Ctrl Pts',(-1.933077639016,-1.28369537222284E-16,
-1.37984607144989));
#456266=CARTESIAN_POINT('Ctrl Pts',(-1.89532807647297,-1.52156718602721E-16,
-1.44943289486579));
#456267=CARTESIAN_POINT('Ctrl Pts',(-1.85404567179292,-5.5994545724509E-16,
-1.5167973757771));
#456268=CARTESIAN_POINT('Ctrl Pts',(-1.80931650950957,-4.71844785465692E-16,
-1.58163386949399));
#456269=CARTESIAN_POINT('Ctrl Pts',(-1.76313966209286,-4.1029866518598E-16,
-1.64856883372233));
#456270=CARTESIAN_POINT('Ctrl Pts',(-1.71329020780722,-3.33757425938898E-17,
-1.71281097695907));
#456271=CARTESIAN_POINT('Ctrl Pts',(-1.66013224533709,-1.17961196366423E-16,
-1.77428904127593));
#456272=CARTESIAN_POINT('Ctrl Pts',(-1.60565559962016,-2.04644951421197E-16,
-1.83729218461563));
#456273=CARTESIAN_POINT('Ctrl Pts',(-1.54770382896436,-9.8490908232494E-17,
-1.89739296998819));
#456274=CARTESIAN_POINT('Ctrl Pts',(-1.48661891555315,-1.04083408558608E-16,
-1.95449269968886));
#456275=CARTESIAN_POINT('Ctrl Pts',(-1.45602320550481,-1.06884534219067E-16,
-1.9830923436304));
#456276=CARTESIAN_POINT('Ctrl Pts',(-1.42464074526194,2.32982061359826E-17,
-2.01093871168437));
#456277=CARTESIAN_POINT('Ctrl Pts',(-1.39251053984076,5.55111512312578E-17,
-2.03801671409802));
#456278=CARTESIAN_POINT('Ctrl Pts',(-1.3768777861536,7.1184161397586E-17,
-2.05119134950803));
#456279=CARTESIAN_POINT('Ctrl Pts',(-1.36106798614324,-3.743924605594E-16,
-2.06418406406673));
#456280=CARTESIAN_POINT('Ctrl Pts',(-1.34508543738201,-3.95516952522712E-16,
-2.07699294275887));
#456281=CARTESIAN_POINT('Ctrl Pts',(-1.33369101195484,-4.1057721931486E-16,
-2.08612476617724));
#456282=CARTESIAN_POINT('Ctrl Pts',(-1.32220764071915,-2.65297351874512E-16,
-2.09516392713986));
#456283=CARTESIAN_POINT('Ctrl Pts',(-1.31065148118413,-2.63677968348475E-16,
-2.10409868877453));
#456284=CARTESIAN_POINT('Ctrl Pts',(-1.24222625606192,-2.54089429700109E-16,
-2.15700234369662));
#456285=CARTESIAN_POINT('Ctrl Pts',(-1.17114186898617,-4.67606722770874E-16,
-2.20633836212491));
#456286=CARTESIAN_POINT('Ctrl Pts',(-1.09779843894241,-4.30211422042248E-16,
-2.25202821416137));
#456287=CARTESIAN_POINT('Ctrl Pts',(-1.02293203288172,-3.92039608050997E-16,
-2.29866681578355));
#456288=CARTESIAN_POINT('Ctrl Pts',(-0.945711177090165,-1.63700498024063E-16,
-2.3415068643473));
#456289=CARTESIAN_POINT('Ctrl Pts',(-0.866514269650375,-9.71445146547012E-17,
-2.3804362849433));
#456290=CARTESIAN_POINT('Ctrl Pts',(-0.786645850745298,-3.00242023568398E-17,
-2.41969578853259));
#456291=CARTESIAN_POINT('Ctrl Pts',(-0.704766937132996,-2.88590153679237E-16,
-2.45497867949436));
#456292=CARTESIAN_POINT('Ctrl Pts',(-0.621228987646033,-3.19189119579733E-16,
-2.48613204577019));
#456293=CARTESIAN_POINT('Ctrl Pts',(-0.581673633799112,-3.33677779296391E-16,
-2.50088321495893));
#456294=CARTESIAN_POINT('Ctrl Pts',(-0.541745863454635,6.25627410058756E-18,
-2.51470792407002));
#456295=CARTESIAN_POINT('Ctrl Pts',(-0.501480960483928,2.77555756156289E-17,
-2.52758639081626));
#456296=CARTESIAN_POINT('Ctrl Pts',(-0.487866421796609,3.50250100518627E-17,
-2.53194091226829));
#456297=CARTESIAN_POINT('Ctrl Pts',(-0.474211239587608,-3.14606215261237E-16,
-2.5361878604183));
#456298=CARTESIAN_POINT('Ctrl Pts',(-0.460523451066253,-3.19189119579733E-16,
-2.54032438870088));
#456299=CARTESIAN_POINT('Ctrl Pts',(-0.372759577575939,-3.48573956596984E-16,
-2.56684713518507));
#456300=CARTESIAN_POINT('Ctrl Pts',(-0.283929367672986,1.93097192062426E-16,
-2.58875295217812));
#456301=CARTESIAN_POINT('Ctrl Pts',(-0.194437403031281,1.11022302462516E-16,
-2.6059343032564));
#456302=CARTESIAN_POINT('Ctrl Pts',(-0.103893064284477,2.79822593000515E-17,
-2.62331769715538));
#456303=CARTESIAN_POINT('Ctrl Pts',(-0.0126704435857078,-3.49772123788992E-16,
-2.63586550789051));
#456304=CARTESIAN_POINT('Ctrl Pts',(0.0788443475852407,-4.44089209850063E-16,
-2.64342393748993));
#456305=CARTESIAN_POINT('Ctrl Pts',(0.170359138756189,-5.38406295911133E-16,
-2.65098236708935));
#456306=CARTESIAN_POINT('Ctrl Pts',(0.262167072908716,-3.46469882950404E-16,
-2.65355201154631));
#456307=CARTESIAN_POINT('Ctrl Pts',(0.353900769383215,-3.60822483003176E-16,
-2.65092764013621));
#456308=CARTESIAN_POINT('Ctrl Pts',(0.385666279468855,-3.65792495978269E-16,
-2.65001887378644));
#456309=CARTESIAN_POINT('Ctrl Pts',(0.417422984221464,-3.15737365300549E-16,
-2.64848679865193));
#456310=CARTESIAN_POINT('Ctrl Pts',(0.449159149942652,-3.60822483003176E-16,
-2.64634069604619));
#456311=CARTESIAN_POINT('Ctrl Pts',(0.478242203475635,-4.02138529283176E-16,
-2.64437400550397));
#456312=CARTESIAN_POINT('Ctrl Pts',(0.507308011629989,2.3581128298129E-16,
-2.64189164976937));
#456313=CARTESIAN_POINT('Ctrl Pts',(0.536347540593685,2.4980018054066E-16,
-2.6389001481074));
#456314=CARTESIAN_POINT('Ctrl Pts',(0.551459749915564,2.57080021352259E-16,
-2.63734336668167));
#456315=CARTESIAN_POINT('Ctrl Pts',(0.566557585451425,-7.49710942941346E-17,
-2.63564938922174));
#456316=CARTESIAN_POINT('Ctrl Pts',(0.581631815384825,-8.32667268468867E-17,
-2.63382058033555));
#456317=CARTESIAN_POINT('Ctrl Pts',(0.670051497316618,-1.31925742596153E-16,
-2.62309348510443));
#456318=CARTESIAN_POINT('Ctrl Pts',(0.757742399593695,-4.64943073742605E-16,
-2.60772302192463));
#456319=CARTESIAN_POINT('Ctrl Pts',(0.844442802535061,-4.44089209850063E-16,
-2.58799378064736));
#456320=CARTESIAN_POINT('Ctrl Pts',(0.936342565858583,-4.21984754840762E-16,
-2.5670813910572));
#456321=CARTESIAN_POINT('Ctrl Pts',(1.02713016079202,-4.81429995614911E-17,
-2.5412720037515));
#456322=CARTESIAN_POINT('Ctrl Pts',(1.11650347932395,-5.55111512312578E-17,
-2.51084435510587));
#456323=CARTESIAN_POINT('Ctrl Pts',(1.19470513303939,-6.19582839423037E-17,
-2.48422016254094));
#456324=CARTESIAN_POINT('Ctrl Pts',(1.27182449504503,-1.67579479506498E-16,
-2.45405903679538));
#456325=CARTESIAN_POINT('Ctrl Pts',(1.34765770122539,-1.94289029309402E-16,
-2.42051198984039));
#456326=CARTESIAN_POINT('Ctrl Pts',(1.38721814572807,-2.08222788883755E-16,
-2.40301126481321));
#456327=CARTESIAN_POINT('Ctrl Pts',(1.42642849848376,-4.25350705594898E-16,
-2.38458854018203));
#456328=CARTESIAN_POINT('Ctrl Pts',(1.46525900971977,-4.44089209850063E-16,
-2.36526192397698));
#456329=CARTESIAN_POINT('Ctrl Pts',(1.484999107099,-4.53615221405509E-16,
-2.35543693651854));
#456330=CARTESIAN_POINT('Ctrl Pts',(1.50464102824796,-4.87876039166925E-16,
-2.34537831594886));
#456331=CARTESIAN_POINT('Ctrl Pts',(1.5241807798872,-4.9960036108132E-16,
-2.33508822707005));
#456332=CARTESIAN_POINT('Ctrl Pts',(1.54114636093401,-5.09780118599735E-16,
-2.3261537564547));
#456333=CARTESIAN_POINT('Ctrl Pts',(1.55803735509877,-7.87150475752769E-16,
-2.31704331667934));
#456334=CARTESIAN_POINT('Ctrl Pts',(1.57482950976773,-7.49400541621981E-16,
-2.30777053426273));
#456335=CARTESIAN_POINT('Ctrl Pts',(1.6591161715088,-5.59918251138288E-16,
-2.2612266636067));
#456336=CARTESIAN_POINT('Ctrl Pts',(1.74102715047747,-4.04388893131409E-16,
-2.21053856448965));
#456337=CARTESIAN_POINT('Ctrl Pts',(1.82025851350983,-3.33066907387547E-16,
-2.15596765860826));
#456338=CARTESIAN_POINT('Ctrl Pts',(1.90298412714173,-2.58599489305927E-16,
-2.09899007419332));
#456339=CARTESIAN_POINT('Ctrl Pts',(1.98278965579871,-3.73079251431402E-16,
-2.03777961061421));
#456340=CARTESIAN_POINT('Ctrl Pts',(2.05931407031973,-3.33066907387547E-16,
-1.97257640891715));
#456341=CARTESIAN_POINT('Ctrl Pts',(2.08396786441214,-3.20176170524201E-16,
-1.95156995863763));
#456342=CARTESIAN_POINT('Ctrl Pts',(2.10828091810247,-2.11292956691504E-16,
-1.93014866511807));
#456343=CARTESIAN_POINT('Ctrl Pts',(2.13224054147413,-1.66533453693773E-16,
-1.90831938598655));
#456344=CARTESIAN_POINT('Ctrl Pts',(2.1496381596241,-1.34032577963915E-16,
-1.89246865841341));
#456345=CARTESIAN_POINT('Ctrl Pts',(2.16685262378074,2.800261672271E-16,
-1.8763995725127));
#456346=CARTESIAN_POINT('Ctrl Pts',(2.18385811644504,2.22044604925031E-16,
-1.86013502292615));
#456347=CARTESIAN_POINT('Ctrl Pts',(2.25541917496481,-2.19484421966021E-17,
-1.79169193763969));
#456348=CARTESIAN_POINT('Ctrl Pts',(2.32334946150237,3.44588198098228E-16,
-1.71973181756775));
#456349=CARTESIAN_POINT('Ctrl Pts',(2.38732344826083,2.22044604925031E-16,
-1.6444973753988));
#456350=CARTESIAN_POINT('Ctrl Pts',(2.4505231820554,1.00984110508486E-16,
-1.57017346722636));
#456351=CARTESIAN_POINT('Ctrl Pts',(2.50986262459353,-7.05684391623025E-17,
-1.49265350674278));
#456352=CARTESIAN_POINT('Ctrl Pts',(2.56500198087084,1.11022302462516E-16,
-1.41212853769079));
#456353=CARTESIAN_POINT('Ctrl Pts',(2.59261215492151,2.01951038681995E-16,
-1.37180691333651));
#456354=CARTESIAN_POINT('Ctrl Pts',(2.61916873567462,-2.90545575616215E-16,
-1.3307311985444));
#456355=CARTESIAN_POINT('Ctrl Pts',(2.64462557919718,-2.77555756156289E-16,
-1.28892185405322));
#456356=CARTESIAN_POINT('Ctrl Pts',(-1.933077639016,-4.11996825544492E-16,
-1.37984607144989));
#456357=CARTESIAN_POINT('Ctrl Pts',(-2.33483719992212,0.046997512537579,
-0.808909857124196));
#456358=CARTESIAN_POINT('Ctrl Pts',(-2.63120278751596,0.146242417143839,
0.799366979810314));
#456359=CARTESIAN_POINT('Ctrl Pts',(-0.877278354639368,0.297734713818778,
2.64988083876425));
#456360=CARTESIAN_POINT('Ctrl Pts',(1.72333502783425,0.454476890024819,
2.1961118038906));
#456361=CARTESIAN_POINT('Ctrl Pts',(2.78243473695495,0.61121906623086,-0.221310618979959));
#456362=CARTESIAN_POINT('Ctrl Pts',(1.58559547981109,0.742590066857593,
-2.08147091584782));
#456363=CARTESIAN_POINT('Ctrl Pts',(0.401815805903339,0.821713675415647,
-2.36781552309403));
#456364=CARTESIAN_POINT('Ctrl Pts',(-0.00016282762489446,0.848589891905021,
-2.36808927594338));
#456365=CARTESIAN_POINT('Origin',(0.,-1.84858989190502,0.));
#456366=CARTESIAN_POINT('',(-1.93106208855765,0.,1.37702479013102));
#456367=CARTESIAN_POINT('Origin',(0.,0.,0.));
#456368=CARTESIAN_POINT('Ctrl Pts',(-1.93106208855765,0.,1.37702479013102));
#456369=CARTESIAN_POINT('Ctrl Pts',(-1.4790123268564,0.0522473920686803,
2.01095394174763));
#456370=CARTESIAN_POINT('Ctrl Pts',(0.0898090403048579,0.15674217620604,
2.78913936379167));
#456371=CARTESIAN_POINT('Ctrl Pts',(2.37789101898706,0.313484352412081,
1.46516877387106));
#456372=CARTESIAN_POINT('Ctrl Pts',(2.53352964655122,0.470226528618122,
-1.16985536842112));
#456373=CARTESIAN_POINT('Ctrl Pts',(1.02001467838193,0.582868447179088,
-2.31145363948848));
#456374=CARTESIAN_POINT('Ctrl Pts',(0.123040243631729,0.643262973671374,
-2.37443199566777));
#456375=CARTESIAN_POINT('Ctrl Pts',(0.00189242379211238,0.651410108094979,
-2.37343051434144));
#456376=CARTESIAN_POINT('Ctrl Pts',(-2.39535560853235,-0.329233991005384,
1.70810875200399));
#456377=CARTESIAN_POINT('Ctrl Pts',(-1.83461758853653,-0.276986598936704,
2.49445620180101));
#456378=CARTESIAN_POINT('Ctrl Pts',(0.111402212112104,-0.172491814799343,
3.45974407432279));
#456379=CARTESIAN_POINT('Ctrl Pts',(2.94961753045639,-0.0157496385933027,
1.81744557087748));
#456380=CARTESIAN_POINT('Ctrl Pts',(3.14267701914353,0.140992537612738,
-1.45112869986083));
#456381=CARTESIAN_POINT('Ctrl Pts',(0.530237091421392,0.297734713818779,
-3.42161261807561));
#456382=CARTESIAN_POINT('Ctrl Pts',(-2.55834405952998,0.454476890024821,
-2.33355215525395));
#456383=CARTESIAN_POINT('Ctrl Pts',(-3.35865124878684,0.61121906623086,
0.840931084698363));
#456384=CARTESIAN_POINT('Ctrl Pts',(-1.15687044439419,0.767961242436902,
3.26350625644717));
#456385=CARTESIAN_POINT('Ctrl Pts',(2.07945874789012,0.924703418642941,
2.76853987221247));
#456386=CARTESIAN_POINT('Ctrl Pts',(3.45658128248051,1.08144559484898,-0.201551325322282));
#456387=CARTESIAN_POINT('Ctrl Pts',(1.74357560709307,1.23818777105502,-2.99143863175781));
#456388=CARTESIAN_POINT('Ctrl Pts',(-1.52824170343262,1.39492994726106,
-3.10696585134584));
#456389=CARTESIAN_POINT('Ctrl Pts',(-3.43377767510254,1.55167212346711,
-0.444838481739954));
#456390=CARTESIAN_POINT('Ctrl Pts',(-2.26950255774756,1.70841429967315,
2.61497556244688));
#456391=CARTESIAN_POINT('Ctrl Pts',(0.923730521087739,1.86515647587919,
3.33698334261355));
#456392=CARTESIAN_POINT('Ctrl Pts',(3.2911386478096,2.02189865208523,1.07570280366772));
#456393=CARTESIAN_POINT('Ctrl Pts',(2.71624608233216,2.17864082829127,-2.1472636142096));
#456394=CARTESIAN_POINT('Ctrl Pts',(-0.286991124867996,2.33538300449731,
-3.450560781959));
#456395=CARTESIAN_POINT('Ctrl Pts',(-3.03365613149575,2.49212518070335,
-1.66903094175379));
#456396=CARTESIAN_POINT('Ctrl Pts',(-3.06820962241996,2.64886735690939,
1.60462451489878));
#456397=CARTESIAN_POINT('Ctrl Pts',(-0.359762533293265,2.80560953311543,
3.44373442996229));
#456398=CARTESIAN_POINT('Ctrl Pts',(2.6703178264213,2.96235170932147,2.20411927030135));
#456399=CARTESIAN_POINT('Ctrl Pts',(3.31310869401662,3.11909388552751,-1.00599263342273));
#456400=CARTESIAN_POINT('Ctrl Pts',(0.993966909026026,3.27583606173356,
-3.31674377806021));
#456401=CARTESIAN_POINT('Ctrl Pts',(-2.21380961171835,3.43257823793959,
-2.66229374567994));
#456402=CARTESIAN_POINT('Ctrl Pts',(-3.4423837489093,3.58932041414564,0.372251560613112));
#456403=CARTESIAN_POINT('Ctrl Pts',(-1.59351869968456,3.74606259035167,
3.07402990583413));
#456404=CARTESIAN_POINT('Ctrl Pts',(1.68011197315232,3.90280476655772,3.02754786397388));
#456405=CARTESIAN_POINT('Ctrl Pts',(3.45142599660708,4.05954694276376,0.274521201611494));
#456406=CARTESIAN_POINT('Ctrl Pts',(2.13768478634502,4.2162891189698,-2.72413174102351));
#456407=CARTESIAN_POINT('Ctrl Pts',(-1.08820815801459,4.37303129517584,
-3.28700278158138));
#456408=CARTESIAN_POINT('Ctrl Pts',(-3.33922505791938,4.52977347138188,
-0.912013904924703));
#456409=CARTESIAN_POINT('Ctrl Pts',(-2.60884382278974,4.68651564758792,
2.27975566396261));
#456410=CARTESIAN_POINT('Ctrl Pts',(0.461684504345609,4.84325782379396,
3.43061028552098));
#456411=CARTESIAN_POINT('Ctrl Pts',(2.22149825342054,4.94775260793132,2.15709966133245));
#456412=CARTESIAN_POINT('Ctrl Pts',(2.64462557919719,5.,1.2889218540532));
#456413=CARTESIAN_POINT('Ctrl Pts',(-2.24059110187412,-0.219489327336923,
1.59774743137966));
#456414=CARTESIAN_POINT('Ctrl Pts',(-1.71608250130982,-0.167241935268243,
2.33328878178322));
#456415=CARTESIAN_POINT('Ctrl Pts',(0.104204488176356,-0.0627471511308821,
3.23620917081242));
#456416=CARTESIAN_POINT('Ctrl Pts',(2.75904202663328,0.093995025075159,
1.70001997187534));
#456417=CARTESIAN_POINT('Ctrl Pts',(2.9396278949461,0.250737201281199,-1.35737092271426));
#456418=CARTESIAN_POINT('Ctrl Pts',(0.495978344380483,0.407479377487241,
-3.20054139719892));
#456419=CARTESIAN_POINT('Ctrl Pts',(-2.39304882953372,0.564221553693281,
-2.18278078469723));
#456420=CARTESIAN_POINT('Ctrl Pts',(-3.14164797724586,0.720963729899322,
0.786598323419274));
#456421=CARTESIAN_POINT('Ctrl Pts',(-1.08212476448077,0.877705906105362,
3.05265032593063));
#456422=CARTESIAN_POINT('Ctrl Pts',(1.94510441399205,1.0344480823114,2.58966383979358));
#456423=CARTESIAN_POINT('Ctrl Pts',(3.23325072771793,1.19119025851744,-0.188529045323978));
#456424=CARTESIAN_POINT('Ctrl Pts',(1.63092276436196,1.34793243472348,-2.79816105643945));
#456425=CARTESIAN_POINT('Ctrl Pts',(-1.42950163642804,1.50467461092953,
-2.90622403435854));
#456426=CARTESIAN_POINT('Ctrl Pts',(-3.21192046694174,1.66141678713557,
-0.416097359576775));
#456427=CARTESIAN_POINT('Ctrl Pts',(-2.12286944721554,1.81815896334161,
2.44602135731598));
#456428=CARTESIAN_POINT('Ctrl Pts',(0.864048068147532,1.97490113954765,
3.12138003974414));
#456429=CARTESIAN_POINT('Ctrl Pts',(3.07849738178723,2.13164331575369,1.00620138470199));
#456430=CARTESIAN_POINT('Ctrl Pts',(2.54074876435687,2.28838549195973,-2.00852839145829));
#456431=CARTESIAN_POINT('Ctrl Pts',(-0.268448558704848,2.44512766816577,
-3.22761921319488));
#456432=CARTESIAN_POINT('Ctrl Pts',(-2.83765087328303,2.60186984437181,
-1.56119444792475));
#456433=CARTESIAN_POINT('Ctrl Pts',(-2.8699718547806,2.75861202057785,1.50094933592518));
#456434=CARTESIAN_POINT('Ctrl Pts',(-0.336518188787201,2.91535419678389,
3.22123391345584));
#456435=CARTESIAN_POINT('Ctrl Pts',(2.49778794419642,3.07209637298993,2.06171058982443));
#456436=CARTESIAN_POINT('Ctrl Pts',(3.09904793798184,3.22883854919597,-0.940995205458836));
#456437=CARTESIAN_POINT('Ctrl Pts',(0.929746466031224,3.38558072540202,
-3.10244815836399));
#456438=CARTESIAN_POINT('Ctrl Pts',(-2.07077483593289,3.54232290160805,
-2.49028230125733));
#456439=CARTESIAN_POINT('Ctrl Pts',(-3.21997050023317,3.6990650778141,0.348200297023759));
#456440=CARTESIAN_POINT('Ctrl Pts',(-1.49056107012472,3.85580725402014,
2.87541608827217));
#456441=CARTESIAN_POINT('Ctrl Pts',(1.57155953119785,4.01254943022618,2.83193726240679));
#456442=CARTESIAN_POINT('Ctrl Pts',(3.22842852611477,4.16929160643222,0.256784320213471));
#456443=CARTESIAN_POINT('Ctrl Pts',(1.99956845398457,4.32603378263826,-2.54812492872817));
#456444=CARTESIAN_POINT('Ctrl Pts',(-1.0178987650724,4.4827759588443,-3.07462873487882));
#456445=CARTESIAN_POINT('Ctrl Pts',(-3.12347691728053,4.63951813505034,
-0.853088465395663));
#456446=CARTESIAN_POINT('Ctrl Pts',(-2.44028579084482,4.79626031125639,
2.13246009775202));
#456447=CARTESIAN_POINT('Ctrl Pts',(0.431854956577303,4.95300248746242,
3.20895772316902));
#456448=CARTESIAN_POINT('Ctrl Pts',(2.07796671263048,5.05749727159978,2.01772892919164));
#456449=CARTESIAN_POINT('Ctrl Pts',(2.47375567929495,5.10974466366846,1.20564430054381));
#456450=CARTESIAN_POINT('Ctrl Pts',(-2.08582659521588,-0.109744663668461,
1.48738611075534));
#456451=CARTESIAN_POINT('Ctrl Pts',(-1.59754741408311,-0.0574972715997809,
2.17212136176543));
#456452=CARTESIAN_POINT('Ctrl Pts',(0.0970067642406067,0.0469975125375791,
3.01267426730204));
#456453=CARTESIAN_POINT('Ctrl Pts',(2.56846652281017,0.20373968874362,1.5825943728732));
#456454=CARTESIAN_POINT('Ctrl Pts',(2.73657877074866,0.360481864949661,
-1.26361314556769));
#456455=CARTESIAN_POINT('Ctrl Pts',(0.461719597339576,0.517224041155702,
-2.97947017632224));
#456456=CARTESIAN_POINT('Ctrl Pts',(-2.22775359953746,0.673966217361742,
-2.03200941414052));
#456457=CARTESIAN_POINT('Ctrl Pts',(-2.92464470570488,0.830708393567783,
0.732265562140186));
#456458=CARTESIAN_POINT('Ctrl Pts',(-1.00737908456736,0.987450569773825,
2.84179439541409));
#456459=CARTESIAN_POINT('Ctrl Pts',(1.81075008009398,1.14419274597986,2.41078780737468));
#456460=CARTESIAN_POINT('Ctrl Pts',(3.00992017295535,1.30093492218591,-0.175506765325674));
#456461=CARTESIAN_POINT('Ctrl Pts',(1.51826992163084,1.45767709839194,-2.60488348112109));
#456462=CARTESIAN_POINT('Ctrl Pts',(-1.33076156942346,1.61441927459799,
-2.70548221737123));
#456463=CARTESIAN_POINT('Ctrl Pts',(-2.99006325878094,1.77116145080402,
-0.387356237413599));
#456464=CARTESIAN_POINT('Ctrl Pts',(-1.97623633668353,1.92790362701007,
2.27706715218508));
#456465=CARTESIAN_POINT('Ctrl Pts',(0.804365615207322,2.08464580321611,
2.90577673687474));
#456466=CARTESIAN_POINT('Ctrl Pts',(2.86585611576487,2.24138797942215,0.936699965736267));
#456467=CARTESIAN_POINT('Ctrl Pts',(2.36525144638157,2.39813015562819,-1.86979316870699));
#456468=CARTESIAN_POINT('Ctrl Pts',(-0.249905992541696,2.55487233183423,
-3.00467764443076));
#456469=CARTESIAN_POINT('Ctrl Pts',(-2.64164561507031,2.71161450804028,
-1.45335795409571));
#456470=CARTESIAN_POINT('Ctrl Pts',(-2.67173408714124,2.86835668424631,
1.39727415695158));
#456471=CARTESIAN_POINT('Ctrl Pts',(-0.313273844281141,3.02509886045236,
2.99873339694938));
#456472=CARTESIAN_POINT('Ctrl Pts',(2.32525806197155,3.18184103665839,1.9193019093475));
#456473=CARTESIAN_POINT('Ctrl Pts',(2.88498718194706,3.33858321286444,-0.875997777494947));
#456474=CARTESIAN_POINT('Ctrl Pts',(0.865526023036425,3.49532538907048,
-2.88815253866777));
#456475=CARTESIAN_POINT('Ctrl Pts',(-1.92774006014744,3.65206756527652,
-2.31827085683471));
#456476=CARTESIAN_POINT('Ctrl Pts',(-2.99755725155704,3.80880974148256,
0.32414903343441));
#456477=CARTESIAN_POINT('Ctrl Pts',(-1.38760344056488,3.9655519176886,2.6768022707102));
#456478=CARTESIAN_POINT('Ctrl Pts',(1.46300708924339,4.12229409389464,2.63632666083971));
#456479=CARTESIAN_POINT('Ctrl Pts',(3.00543105562245,4.27903627010068,0.239047438815444));
#456480=CARTESIAN_POINT('Ctrl Pts',(1.86145212162413,4.43577844630672,-2.37211811643283));
#456481=CARTESIAN_POINT('Ctrl Pts',(-0.947589372130199,4.59252062251276,
-2.86225468817626));
#456482=CARTESIAN_POINT('Ctrl Pts',(-2.90772877664167,4.74926279871881,
-0.794163025866617));
#456483=CARTESIAN_POINT('Ctrl Pts',(-2.2717277588999,4.90600497492485,1.98516453154143));
#456484=CARTESIAN_POINT('Ctrl Pts',(0.402025408808995,5.06274715113088,
2.98730516081707));
#456485=CARTESIAN_POINT('Ctrl Pts',(1.93443517184043,5.16724193526824,1.87835819705082));
#456486=CARTESIAN_POINT('Ctrl Pts',(2.3028857793927,5.21948932733692,1.12236674703442));
#456487=CARTESIAN_POINT('Ctrl Pts',(-1.93106208855765,0.,1.37702479013102));
#456488=CARTESIAN_POINT('Ctrl Pts',(-1.4790123268564,0.0522473920686803,
2.01095394174763));
#456489=CARTESIAN_POINT('Ctrl Pts',(0.0898090403048579,0.15674217620604,
2.78913936379167));
#456490=CARTESIAN_POINT('Ctrl Pts',(2.37789101898706,0.313484352412081,
1.46516877387106));
#456491=CARTESIAN_POINT('Ctrl Pts',(2.53352964655122,0.470226528618122,
-1.16985536842112));
#456492=CARTESIAN_POINT('Ctrl Pts',(0.427460850298667,0.626968704824163,
-2.75839895544555));
#456493=CARTESIAN_POINT('Ctrl Pts',(-2.06245836954121,0.783710881030204,
-1.88123804358381));
#456494=CARTESIAN_POINT('Ctrl Pts',(-2.7076414341639,0.940453057236244,
0.677932800861099));
#456495=CARTESIAN_POINT('Ctrl Pts',(-0.932633404653946,1.09719523344229,
2.63093846489754));
#456496=CARTESIAN_POINT('Ctrl Pts',(1.67639574619592,1.25393740964833,2.23191177495579));
#456497=CARTESIAN_POINT('Ctrl Pts',(2.78658961819278,1.41067958585437,-0.162484485327371));
#456498=CARTESIAN_POINT('Ctrl Pts',(1.40561707889972,1.56742176206041,-2.41160590580272));
#456499=CARTESIAN_POINT('Ctrl Pts',(-1.23202150241888,1.72416393826645,
-2.50474040038392));
#456500=CARTESIAN_POINT('Ctrl Pts',(-2.76820605062014,1.88090611447249,
-0.358615115250419));
#456501=CARTESIAN_POINT('Ctrl Pts',(-1.82960322615152,2.03764829067853,
2.10811294705418));
#456502=CARTESIAN_POINT('Ctrl Pts',(0.744683162267116,2.19439046688457,
2.69017343400533));
#456503=CARTESIAN_POINT('Ctrl Pts',(2.65321484974249,2.35113264309061,0.867198546770537));
#456504=CARTESIAN_POINT('Ctrl Pts',(2.18975412840629,2.50787481929665,-1.73105794595568));
#456505=CARTESIAN_POINT('Ctrl Pts',(-0.231363426378548,2.66461699550269,
-2.78173607566664));
#456506=CARTESIAN_POINT('Ctrl Pts',(-2.44564035685759,2.82135917170873,
-1.34552146026667));
#456507=CARTESIAN_POINT('Ctrl Pts',(-2.47349631950189,2.97810134791478,
1.29359897797797));
#456508=CARTESIAN_POINT('Ctrl Pts',(-0.29002949977508,3.13484352412081,
2.77623288044292));
#456509=CARTESIAN_POINT('Ctrl Pts',(2.15272817974667,3.29158570032686,1.77689322887057));
#456510=CARTESIAN_POINT('Ctrl Pts',(2.67092642591228,3.44832787653289,-0.811000349531056));
#456511=CARTESIAN_POINT('Ctrl Pts',(0.801305580041626,3.60507005273894,
-2.67385691897155));
#456512=CARTESIAN_POINT('Ctrl Pts',(-1.78470528436199,3.76181222894497,
-2.1462594124121));
#456513=CARTESIAN_POINT('Ctrl Pts',(-2.77514400288091,3.91855440515103,
0.300097769845058));
#456514=CARTESIAN_POINT('Ctrl Pts',(-1.28464581100504,4.07529658135705,
2.47818845314823));
#456515=CARTESIAN_POINT('Ctrl Pts',(1.35445464728892,4.2320387575631,2.44071605927262));
#456516=CARTESIAN_POINT('Ctrl Pts',(2.78243358513013,4.38878093376914,0.221310557417421));
#456517=CARTESIAN_POINT('Ctrl Pts',(1.72333578926369,4.54552310997518,-2.19611130413749));
#456518=CARTESIAN_POINT('Ctrl Pts',(-0.877279979188005,4.70226528618122,
-2.6498806414737));
#456519=CARTESIAN_POINT('Ctrl Pts',(-2.69198063600282,4.85900746238726,
-0.735237586337578));
#456520=CARTESIAN_POINT('Ctrl Pts',(-2.10316972695498,5.01574963859331,
1.83786896533084));
#456521=CARTESIAN_POINT('Ctrl Pts',(0.372195861040687,5.17249181479935,
2.76565259846512));
#456522=CARTESIAN_POINT('Ctrl Pts',(1.79090363105037,5.27698659893671,1.73898746491001));
#456523=CARTESIAN_POINT('Ctrl Pts',(2.13201587949046,5.32923399100539,1.03908919352504));
#456524=CARTESIAN_POINT('',(2.64462557919717,5.,1.28892185405323));
#456525=CARTESIAN_POINT('Ctrl Pts',(-1.93307880200417,5.,1.37984525234447));
#456526=CARTESIAN_POINT('Ctrl Pts',(-1.89532923114376,5.,1.44943208196965));
#456527=CARTESIAN_POINT('Ctrl Pts',(-1.8540467895405,5.,1.51679658079351));
#456528=CARTESIAN_POINT('Ctrl Pts',(-1.80931755641146,5.,1.58163310600374));
#456529=CARTESIAN_POINT('Ctrl Pts',(-1.76314072863898,5.,1.64856796825283));
#456530=CARTESIAN_POINT('Ctrl Pts',(-1.71329127262828,5.,1.71281003478393));
#456531=CARTESIAN_POINT('Ctrl Pts',(-1.66013329288395,5.,1.7742880449691));
#456532=CARTESIAN_POINT('Ctrl Pts',(-1.60565658732334,5.,1.83729118157092));
#456533=CARTESIAN_POINT('Ctrl Pts',(-1.54770473511596,5.,1.8973919794258));
#456534=CARTESIAN_POINT('Ctrl Pts',(-1.48661972537529,5.,1.95449173807213));
#456535=CARTESIAN_POINT('Ctrl Pts',(-1.45602391706679,5.,1.98309144326039));
#456536=CARTESIAN_POINT('Ctrl Pts',(-1.42464135228175,5.,2.01093787423408));
#456537=CARTESIAN_POINT('Ctrl Pts',(-1.39251103708368,5.,2.03801594084573));
#456538=CARTESIAN_POINT('Ctrl Pts',(-1.37687840864276,5.,2.05119045692593));
#456539=CARTESIAN_POINT('Ctrl Pts',(-1.36106873668559,5.,2.06418305661536));
#456540=CARTESIAN_POINT('Ctrl Pts',(-1.34508631875706,5.,2.07699182491987));
#456541=CARTESIAN_POINT('Ctrl Pts',(-1.33369143914598,5.,2.08612400838853));
#456542=CARTESIAN_POINT('Ctrl Pts',(-1.32220760631118,5.,2.09516352299594));
#456543=CARTESIAN_POINT('Ctrl Pts',(-1.31065097934111,5.,2.10409863074976));
#456544=CARTESIAN_POINT('Ctrl Pts',(-1.24222560571871,5.,2.15700230999759));
#456545=CARTESIAN_POINT('Ctrl Pts',(-1.17114106324171,5.,2.20633836739357));
#456546=CARTESIAN_POINT('Ctrl Pts',(-1.09779747805985,5.,2.25202826990409));
#456547=CARTESIAN_POINT('Ctrl Pts',(-1.02293085554802,5.,2.29866695923699));
#456548=CARTESIAN_POINT('Ctrl Pts',(-0.945709779919864,5.,2.34150710161237));
#456549=CARTESIAN_POINT('Ctrl Pts',(-0.866512657585552,5.,2.38043661881683));
#456550=CARTESIAN_POINT('Ctrl Pts',(-0.786643980132719,5.,2.41969624039592));
#456551=CARTESIAN_POINT('Ctrl Pts',(-0.70476481087952,5.,2.4549792480358));
#456552=CARTESIAN_POINT('Ctrl Pts',(-0.62122661766354,5.,2.48613272617783));
#456553=CARTESIAN_POINT('Ctrl Pts',(-0.581671214473811,5.,2.50088392369876));
#456554=CARTESIAN_POINT('Ctrl Pts',(-0.541743398700346,5.,2.51470866315734));
#456555=CARTESIAN_POINT('Ctrl Pts',(-0.501478455000533,5.,2.52758716199342));
#456556=CARTESIAN_POINT('Ctrl Pts',(-0.487863882992778,5.,2.53194170054842));
#456557=CARTESIAN_POINT('Ctrl Pts',(-0.474208668049177,5.,2.53618866564346));
#456558=CARTESIAN_POINT('Ctrl Pts',(-0.460520846856072,5.,2.54032521086352));
#456559=CARTESIAN_POINT('Ctrl Pts',(-0.372756764672366,5.,2.56684806570853));
#456560=CARTESIAN_POINT('Ctrl Pts',(-0.283926366055009,5.,2.5887539852999));
#456561=CARTESIAN_POINT('Ctrl Pts',(-0.19443424169612,5.,2.60593542971511));
#456562=CARTESIAN_POINT('Ctrl Pts',(-0.103889636373118,5.,2.62331893820371));
#456563=CARTESIAN_POINT('Ctrl Pts',(-0.0126667771947791,5.,2.63586684285107));
#456564=CARTESIAN_POINT('Ctrl Pts',(0.078848213731232,5.,2.64342534156938));
#456565=CARTESIAN_POINT('Ctrl Pts',(0.170363204657243,5.,2.65098384028769));
#456566=CARTESIAN_POINT('Ctrl Pts',(0.262171299865505,5.,2.65355352908114));
#456567=CARTESIAN_POINT('Ctrl Pts',(0.353905107892403,5.,2.65092917282106));
#456568=CARTESIAN_POINT('Ctrl Pts',(0.385670645239163,5.,2.65002041204263));
#456569=CARTESIAN_POINT('Ctrl Pts',(0.417427371319863,5.,2.64848833942243));
#456570=CARTESIAN_POINT('Ctrl Pts',(0.449163552816194,5.,2.64634223644399));
#456571=CARTESIAN_POINT('Ctrl Pts',(0.478246692955225,5.,2.64437554068124));
#456572=CARTESIAN_POINT('Ctrl Pts',(0.5073125829666,5.,2.64189317474323));
#456573=CARTESIAN_POINT('Ctrl Pts',(0.536352189258467,5.,2.63890165807019));
#456574=CARTESIAN_POINT('Ctrl Pts',(0.55146429954055,5.,2.63734488318077));
#456575=CARTESIAN_POINT('Ctrl Pts',(0.566562034763081,5.,2.63565091351987));
#456576=CARTESIAN_POINT('Ctrl Pts',(0.581636163657774,5.,2.63382211363912));
#456577=CARTESIAN_POINT('Ctrl Pts',(0.670055756250796,5.,2.62309501016801));
#456578=CARTESIAN_POINT('Ctrl Pts',(0.757746531289113,5.,2.60772452781098));
#456579=CARTESIAN_POINT('Ctrl Pts',(0.844446778749971,5.,2.58799525961142));
#456580=CARTESIAN_POINT('Ctrl Pts',(0.936346421350173,5.,2.56708283145346));
#456581=CARTESIAN_POINT('Ctrl Pts',(1.0271338627505,5.,2.54127339218079));
#456582=CARTESIAN_POINT('Ctrl Pts',(1.11650700532631,5.,2.51084568220488));
#456583=CARTESIAN_POINT('Ctrl Pts',(1.19470850508015,5.,2.48422143597595));
#456584=CARTESIAN_POINT('Ctrl Pts',(1.27182769593864,5.,2.45406024939045));
#456585=CARTESIAN_POINT('Ctrl Pts',(1.34766072047862,5.,2.42051313701281));
#456586=CARTESIAN_POINT('Ctrl Pts',(1.38722105531367,5.,2.40301238445205));
#456587=CARTESIAN_POINT('Ctrl Pts',(1.42643129580676,5.,2.38458963173364));
#456588=CARTESIAN_POINT('Ctrl Pts',(1.46526169315625,5.,2.3652629872301));
#456589=CARTESIAN_POINT('Ctrl Pts',(1.48500186360994,5.,2.35543792019914));
#456590=CARTESIAN_POINT('Ctrl Pts',(1.50464385611093,5.,2.34537921690229));
#456591=CARTESIAN_POINT('Ctrl Pts',(1.52418367742757,5.,2.33508904222946));
#456592=CARTESIAN_POINT('Ctrl Pts',(1.54114915715179,5.,2.32615458234155));
#456593=CARTESIAN_POINT('Ctrl Pts',(1.55804005009276,5.,2.31704415436288));
#456594=CARTESIAN_POINT('Ctrl Pts',(1.57483210399388,5.,2.30777138474885));
#456595=CARTESIAN_POINT('Ctrl Pts',(1.65911847268188,5.,2.26122746087573));
#456596=CARTESIAN_POINT('Ctrl Pts',(1.74102915795926,5.,2.21053931269157));
#456597=CARTESIAN_POINT('Ctrl Pts',(1.82026023750243,5.,2.15596836522314));
#456598=CARTESIAN_POINT('Ctrl Pts',(1.90298562056131,5.,2.09899069232961));
#456599=CARTESIAN_POINT('Ctrl Pts',(1.98279092512795,5.,2.03778014173156));
#456600=CARTESIAN_POINT('Ctrl Pts',(2.05931513335921,5.,1.97257685889539));
#456601=CARTESIAN_POINT('Ctrl Pts',(2.08396884136544,5.,1.95157039919793));
#456602=CARTESIAN_POINT('Ctrl Pts',(2.10828181135941,5.,1.93014909753088));
#456603=CARTESIAN_POINT('Ctrl Pts',(2.13224135383482,5.,1.90831981165407));
#456604=CARTESIAN_POINT('Ctrl Pts',(2.14963896322531,5.,1.89246903364578));
#456605=CARTESIAN_POINT('Ctrl Pts',(2.16685341904675,5.,1.8763998967844));
#456606=CARTESIAN_POINT('Ctrl Pts',(2.18385890387661,5.,1.86013529589314));
#456607=CARTESIAN_POINT('Ctrl Pts',(2.25541977559558,5.,1.79169214184112));
#456608=CARTESIAN_POINT('Ctrl Pts',(2.32334989974494,5.,1.71973196190852));
#456609=CARTESIAN_POINT('Ctrl Pts',(2.38732375899673,5.,1.64449747278477));
#456610=CARTESIAN_POINT('Ctrl Pts',(2.45052346277645,5.,1.57017340538836));
#456611=CARTESIAN_POINT('Ctrl Pts',(2.50986289761011,5.,1.49265328857437));
#456612=CARTESIAN_POINT('Ctrl Pts',(2.56500227712659,5.,1.41212817082369));
#456613=CARTESIAN_POINT('Ctrl Pts',(2.59261233427658,5.,1.37180665972577));
#456614=CARTESIAN_POINT('Ctrl Pts',(2.61916881569582,5.,1.33073106712064));
#456615=CARTESIAN_POINT('Ctrl Pts',(2.64462557919719,5.,1.2889218540532));
#456616=CARTESIAN_POINT('Ctrl Pts',(2.64767078191736,2.08166817117217E-17,
1.29195911160569));
#456617=CARTESIAN_POINT('Ctrl Pts',(2.59777293643844,-9.41002177091934E-18,
1.37498592169266));
#456618=CARTESIAN_POINT('Ctrl Pts',(2.54371157748951,-6.47715074628022E-17,
1.45513970804844));
#456619=CARTESIAN_POINT('Ctrl Pts',(2.48549620893604,0.,1.53206089300545));
#456620=CARTESIAN_POINT('Ctrl Pts',(2.42718272400871,7.79025300962201E-17,
1.60911172118088));
#456621=CARTESIAN_POINT('Ctrl Pts',(2.36470052429476,1.68964082133378E-16,
1.68291956022001));
#456622=CARTESIAN_POINT('Ctrl Pts',(2.29842841323133,1.04083408558608E-16,
1.753333246675));
#456623=CARTESIAN_POINT('Ctrl Pts',(2.22837578437846,3.55015922753236E-17,
1.82776370866335));
#456624=CARTESIAN_POINT('Ctrl Pts',(2.1540876478833,-1.73068786219787E-16,
1.89840261978313));
#456625=CARTESIAN_POINT('Ctrl Pts',(2.07598043274033,-1.38777878078145E-16,
1.96501840927444));
#456626=CARTESIAN_POINT('Ctrl Pts',(2.04180852611527,-1.23775605766176E-16,
1.99416281717689));
#456627=CARTESIAN_POINT('Ctrl Pts',(2.00690532118568,-1.61221863714727E-16,
2.02253643282966));
#456628=CARTESIAN_POINT('Ctrl Pts',(1.97130468257589,-2.0122792321331E-16,
2.05011625538801));
#456629=CARTESIAN_POINT('Ctrl Pts',(1.9466006592944,-2.28988959639827E-16,
2.06925446765574));
#456630=CARTESIAN_POINT('Ctrl Pts',(1.92156079295665,3.52147159119889E-16,
2.0880104013613));
#456631=CARTESIAN_POINT('Ctrl Pts',(1.89619633295332,3.60822483003176E-16,
2.10637570990819));
#456632=CARTESIAN_POINT('Ctrl Pts',(1.88438018844951,3.6486392053462E-16,
2.11493126912839));
#456633=CARTESIAN_POINT('Ctrl Pts',(1.87250046861909,3.5548778546167E-16,
2.12339705091612));
#456634=CARTESIAN_POINT('Ctrl Pts',(1.86056161129017,3.60822483003176E-16,
2.13177039141816));
#456635=CARTESIAN_POINT('Ctrl Pts',(1.7820029969632,3.95925209769072E-16,
2.18686762635492));
#456636=CARTESIAN_POINT('Ctrl Pts',(1.70084278960875,-6.39194753652185E-16,
2.23799746638749));
#456637=CARTESIAN_POINT('Ctrl Pts',(1.61744804048977,-5.68989300120393E-16,
2.2850133461233));
#456638=CARTESIAN_POINT('Ctrl Pts',(1.53432414409267,-4.99011862601365E-16,
2.33187652584943));
#456639=CARTESIAN_POINT('Ctrl Pts',(1.4489792272881,2.66553321917947E-16,
2.37465270447628));
#456640=CARTESIAN_POINT('Ctrl Pts',(1.36175994557255,3.7470027081099E-16,
2.41314817623965));
#456641=CARTESIAN_POINT('Ctrl Pts',(1.27604626988848,4.80980353853544E-16,
2.45097912734508));
#456642=CARTESIAN_POINT('Ctrl Pts',(1.18852150214909,2.31652411642962E-17,
2.48467602422174));
#456643=CARTESIAN_POINT('Ctrl Pts',(1.09951206593735,9.71445146547012E-17,
2.514005137696));
#456644=CARTESIAN_POINT('Ctrl Pts',(1.05865205862629,1.31104887670592E-16,
2.52746874157878));
#456645=CARTESIAN_POINT('Ctrl Pts',(1.01747923206645,3.9815101041052E-16,
2.54001121457231));
#456646=CARTESIAN_POINT('Ctrl Pts',(0.976025735328773,4.02455846426619E-16,
2.55160621007744));
#456647=CARTESIAN_POINT('Ctrl Pts',(0.957564524483282,4.04372994353883E-16,
2.55677001225624));
#456648=CARTESIAN_POINT('Ctrl Pts',(0.939047654610198,2.79685920519915E-17,
2.56174586500462));
#456649=CARTESIAN_POINT('Ctrl Pts',(0.920478007731592,2.77555756156289E-17,
2.56653128470133));
#456650=CARTESIAN_POINT('Ctrl Pts',(0.907358149967187,2.76050748891031E-17,
2.56991228737597));
#456651=CARTESIAN_POINT('Ctrl Pts',(0.894221412269896,4.16935637140537E-16,
2.5731957889532));
#456652=CARTESIAN_POINT('Ctrl Pts',(0.881069062795557,4.16333634234434E-16,
2.57638126889446));
#456653=CARTESIAN_POINT('Ctrl Pts',(0.791883790902668,4.12251489598156E-16,
2.59798181222135));
#456654=CARTESIAN_POINT('Ctrl Pts',(0.701977238002251,-8.43023025612678E-17,
2.6150803310287));
#456655=CARTESIAN_POINT('Ctrl Pts',(0.611665199798742,5.55111512312578E-17,
2.62750524997846));
#456656=CARTESIAN_POINT('Ctrl Pts',(0.523980164752349,1.91257701078017E-16,
2.6395687519792));
#456657=CARTESIAN_POINT('Ctrl Pts',(0.435912140235754,-1.98170145761692E-17,
2.64722656595151));
#456658=CARTESIAN_POINT('Ctrl Pts',(0.347753491767775,0.,2.65027380970596));
#456659=CARTESIAN_POINT('Ctrl Pts',(0.26115622397153,1.94660347906529E-17,
2.65326708362781));
#456660=CARTESIAN_POINT('Ctrl Pts',(0.174470883311766,-9.45420770462548E-17,
2.65181170424695));
#456661=CARTESIAN_POINT('Ctrl Pts',(0.0879878877595678,-2.22044604925031E-16,
2.64566633498951));
#456662=CARTESIAN_POINT('Ctrl Pts',(0.0366511445548616,-2.97730749812473E-16,
2.64201841274245));
#456663=CARTESIAN_POINT('Ctrl Pts',(-0.0146139987793563,-2.74135710604959E-16,
2.63671681157407));
#456664=CARTESIAN_POINT('Ctrl Pts',(-0.0657434791662867,-3.33066907387547E-16,
2.62978938315714));
#456665=CARTESIAN_POINT('Ctrl Pts',(-0.0799608240973768,-3.49453640550479E-16,
2.62786310425613));
#456666=CARTESIAN_POINT('Ctrl Pts',(-0.0941694681167345,1.46489281919524E-16,
2.62581081298278));
#456667=CARTESIAN_POINT('Ctrl Pts',(-0.108362279338616,1.38777878078145E-16,
2.62363393548456));
#456668=CARTESIAN_POINT('Ctrl Pts',(-0.195237834838755,9.15756373146707E-17,
2.61030906002775));
#456669=CARTESIAN_POINT('Ctrl Pts',(-0.281234873934964,-1.80842283591821E-16,
2.59236560928012));
#456670=CARTESIAN_POINT('Ctrl Pts',(-0.366067255626018,-1.11022302462516E-16,
2.57003468112992));
#456671=CARTESIAN_POINT('Ctrl Pts',(-0.452591139793857,-3.98101563526326E-17,
2.54725848880674));
#456672=CARTESIAN_POINT('Ctrl Pts',(-0.537904334660485,3.59163319751851E-16,
2.5199176109006));
#456673=CARTESIAN_POINT('Ctrl Pts',(-0.621681621332169,4.16333634234434E-16,
2.48820833141206));
#456674=CARTESIAN_POINT('Ctrl Pts',(-0.704713214603355,4.72995081362776E-16,
2.45678129310593));
#456675=CARTESIAN_POINT('Ctrl Pts',(-0.786236851551895,-7.23320616115926E-17,
2.42106258564705));
#456676=CARTESIAN_POINT('Ctrl Pts',(-0.865902984875024,-8.32667268468867E-17,
2.38120496126432));
#456677=CARTESIAN_POINT('Ctrl Pts',(-0.901639793419379,-8.81718229236015E-17,
2.36332554083581));
#456678=CARTESIAN_POINT('Ctrl Pts',(-0.937002314170247,2.77664426612253E-16,
2.34461280846694));
#456679=CARTESIAN_POINT('Ctrl Pts',(-0.971956223286635,3.05311331771918E-16,
2.32507856243581));
#456680=CARTESIAN_POINT('Ctrl Pts',(-0.992272043074096,3.21380193799183E-16,
2.31372491896403));
#456681=CARTESIAN_POINT('Ctrl Pts',(-1.01244979378511,3.7665599969535E-16,
2.30209373598401));
#456682=CARTESIAN_POINT('Ctrl Pts',(-1.03248242996565,3.88578058618805E-16,
2.29018717062679));
#456683=CARTESIAN_POINT('Ctrl Pts',(-1.04555838107585,3.96359973001472E-16,
2.28241536939711));
#456684=CARTESIAN_POINT('Ctrl Pts',(-1.05856453943241,7.49772963088282E-17,
2.2745309510009));
#456685=CARTESIAN_POINT('Ctrl Pts',(-1.07149704589891,8.32667268468867E-17,
2.26653625180142));
#456686=CARTESIAN_POINT('Ctrl Pts',(-1.14591162693116,1.30964711926809E-16,
2.22053417223948));
#456687=CARTESIAN_POINT('Ctrl Pts',(-1.21791517776447,-5.54854112154195E-17,
2.17086906248028));
#456688=CARTESIAN_POINT('Ctrl Pts',(-1.28718220994981,0.,2.11770866201185));
#456689=CARTESIAN_POINT('Ctrl Pts',(-1.35260428900227,5.24054639598309E-17,
2.06749914946049));
#456690=CARTESIAN_POINT('Ctrl Pts',(-1.41558545623252,4.02940859333988E-16,
2.01417086704383));
#456691=CARTESIAN_POINT('Ctrl Pts',(-1.47581496564193,3.33066907387547E-16,
1.95784111287787));
#456692=CARTESIAN_POINT('Ctrl Pts',(-1.49258172621148,3.1361531573717E-16,
1.94215997068854));
#456693=CARTESIAN_POINT('Ctrl Pts',(-1.50913500506103,1.49129398006594E-16,
1.92624611129061));
#456694=CARTESIAN_POINT('Ctrl Pts',(-1.5254675200324,1.66533453693773E-16,
1.91010182088324));
#456695=CARTESIAN_POINT('Ctrl Pts',(-1.54179187160703,1.83928810401539E-16,
1.8939655997933));
#456696=CARTESIAN_POINT('Ctrl Pts',(-1.5578994091293,2.07719017048048E-16,
1.87759507106596));
#456697=CARTESIAN_POINT('Ctrl Pts',(-1.57376072394509,2.22044604925031E-16,
1.86101591094124));
#456698=CARTESIAN_POINT('Ctrl Pts',(-1.63177025543134,2.74437527621558E-16,
1.80038100630439));
#456699=CARTESIAN_POINT('Ctrl Pts',(-1.6865409807442,-5.20802644289233E-17,
1.73690974699413));
#456700=CARTESIAN_POINT('Ctrl Pts',(-1.73775514238363,-1.11022302462516E-16,
1.67073873704775));
#456701=CARTESIAN_POINT('Ctrl Pts',(-1.78752738553671,-1.68304846099581E-16,
1.60643075091055));
#456702=CARTESIAN_POINT('Ctrl Pts',(-1.83394083805679,4.77778439695772E-16,
1.53957230095707));
#456703=CARTESIAN_POINT('Ctrl Pts',(-1.87665805183407,4.9960036108132E-16,
1.4702714467312));
#456704=CARTESIAN_POINT('Ctrl Pts',(-1.89552518062833,5.09238559945739E-16,
1.43966298642645));
#456705=CARTESIAN_POINT('Ctrl Pts',(-1.9136706201995,1.36541150579267E-17,
1.40857789095612));
#456706=CARTESIAN_POINT('Ctrl Pts',(-1.93106208855765,0.,1.37702479013102));
#456707=CARTESIAN_POINT('Ctrl Pts',(2.64462557919719,5.,1.2889218540532));
#456708=CARTESIAN_POINT('Ctrl Pts',(2.22149825342054,4.94775260793132,2.15709966133245));
#456709=CARTESIAN_POINT('Ctrl Pts',(1.34159137888307,4.89550521586264,2.79385497342672));
#456710=CARTESIAN_POINT('Ctrl Pts',(0.389883220425111,4.84325782379396,
2.92042352588079));
#456711=CARTESIAN_POINT('Ctrl Pts',(-0.561824938032845,4.79101043172528,
3.04699207833485));
#456712=CARTESIAN_POINT('Ctrl Pts',(-1.58533438041129,4.7387630396566,2.66337387114873));
#456713=CARTESIAN_POINT('Ctrl Pts',(-2.21881930745545,4.68651564758792,
1.93960317274112));
#456714=CARTESIAN_POINT('Ctrl Pts',(-2.85230423449962,4.63426825551924,
1.21583247433351));
#456715=CARTESIAN_POINT('Ctrl Pts',(-3.0957646462095,4.58202086345056,0.151909284704409));
#456716=CARTESIAN_POINT('Ctrl Pts',(-2.84232536874697,4.52977347138188,
-0.775883789552923));
#456717=CARTESIAN_POINT('Ctrl Pts',(-2.58888609128445,4.4775260793132,-1.70367686381026));
#456718=CARTESIAN_POINT('Ctrl Pts',(-1.83854712464952,4.42527868724452,
-2.49533982269582));
#456719=CARTESIAN_POINT('Ctrl Pts',(-0.925728817272116,4.37303129517584,
-2.79735946204562));
#456720=CARTESIAN_POINT('Ctrl Pts',(-0.629563874908174,4.35607956914709,
-2.89535007897113));
#456721=CARTESIAN_POINT('Ctrl Pts',(-0.316294968976919,4.33912784311834,
-2.94179665675882));
#456722=CARTESIAN_POINT('Ctrl Pts',(-0.00235626413880502,4.3221761170896,
-2.93955723260335));
#456723=CARTESIAN_POINT('Origin',(3.,5.,0.));
#456724=CARTESIAN_POINT('Origin',(0.,5.,0.));
#456725=CARTESIAN_POINT('',(-1.71450551880629E-16,5.,-1.4));
#456726=CARTESIAN_POINT('Origin',(0.,5.,0.));
#456727=CARTESIAN_POINT('Origin',(0.,0.,0.));
#456728=CARTESIAN_POINT('Origin',(-5.65994024385247E-16,16.9,0.));
#456729=CARTESIAN_POINT('',(2.08623127625816,16.9,-2.15132589821367));
#456730=CARTESIAN_POINT('',(-3.67394039744206E-16,16.9,-3.));
#456731=CARTESIAN_POINT('Origin',(0.,16.9,0.));
#456732=CARTESIAN_POINT('Ctrl Pts',(2.08484969764298,16.9,-2.14815125844468));
#456733=CARTESIAN_POINT('Ctrl Pts',(2.04033184400282,16.9,-2.18402695258335));
#456734=CARTESIAN_POINT('Ctrl Pts',(1.99479799836031,16.9,-2.21871156426885));
#456735=CARTESIAN_POINT('Ctrl Pts',(1.94829228233076,16.9,-2.25214199615432));
#456736=CARTESIAN_POINT('Ctrl Pts',(1.93304371715383,16.9,-2.26310336097181));
#456737=CARTESIAN_POINT('Ctrl Pts',(1.91769066004217,16.9,-2.27392984482344));
#456738=CARTESIAN_POINT('Ctrl Pts',(1.90223464967274,16.9,-2.28461908837391));
#456739=CARTESIAN_POINT('Ctrl Pts',(1.8913609280757,16.9,-2.29213926050583));
#456740=CARTESIAN_POINT('Ctrl Pts',(1.88043666951372,16.9,-2.2995911555075));
#456741=CARTESIAN_POINT('Ctrl Pts',(1.86947174693695,16.9,-2.30696784701081));
#456742=CARTESIAN_POINT('Ctrl Pts',(1.78751170222814,16.9,-2.36210676488104));
#456743=CARTESIAN_POINT('Ctrl Pts',(1.70314050175845,16.9,-2.41314579558716));
#456744=CARTESIAN_POINT('Ctrl Pts',(1.61662095764565,16.9,-2.45984009817923));
#456745=CARTESIAN_POINT('Ctrl Pts',(1.53131758125062,16.9,-2.50587803920584));
#456746=CARTESIAN_POINT('Ctrl Pts',(1.44392509555319,16.9,-2.54769287785561));
#456747=CARTESIAN_POINT('Ctrl Pts',(1.35467911748674,16.9,-2.58500289820093));
#456748=CARTESIAN_POINT('Ctrl Pts',(1.26823404221274,16.9,-2.62114197793429));
#456749=CARTESIAN_POINT('Ctrl Pts',(1.1800493652205,16.9,-2.65305469538287));
#456750=CARTESIAN_POINT('Ctrl Pts',(1.09033375493529,16.9,-2.6804373720982));
#456751=CARTESIAN_POINT('Ctrl Pts',(1.01566330819408,16.9,-2.70322801797135));
#456752=CARTESIAN_POINT('Ctrl Pts',(0.939932095011573,16.9,-2.72287985795654));
#456753=CARTESIAN_POINT('Ctrl Pts',(0.863261863496793,16.9,-2.73919020059434));
#456754=CARTESIAN_POINT('',(-2.95306835703349,16.9,-0.516208692970735));
#456755=CARTESIAN_POINT('Ctrl Pts',(-2.312781279227,16.9,-1.71040874167461));
#456756=CARTESIAN_POINT('Ctrl Pts',(-2.36394961038129,16.9,-1.65422188238401));
#456757=CARTESIAN_POINT('Ctrl Pts',(-2.41264488535713,16.9,-1.59599660500464));
#456758=CARTESIAN_POINT('Ctrl Pts',(-2.45869800638489,16.9,-1.53582544180072));
#456759=CARTESIAN_POINT('Ctrl Pts',(-2.5162098854388,16.9,-1.4606827243586));
#456760=CARTESIAN_POINT('Ctrl Pts',(-2.56960306603727,16.9,-1.38250657480199));
#456761=CARTESIAN_POINT('Ctrl Pts',(-2.61891115144116,16.9,-1.30168621892116));
#456762=CARTESIAN_POINT('Ctrl Pts',(-2.6576091123471,16.9,-1.23825680472547));
#456763=CARTESIAN_POINT('Ctrl Pts',(-2.6937902591549,16.9,-1.17319770675496));
#456764=CARTESIAN_POINT('Ctrl Pts',(-2.72745504689701,16.9,-1.10668186268529));
#456765=CARTESIAN_POINT('Ctrl Pts',(-2.73624314508487,16.9,-1.08931808860744));
#456766=CARTESIAN_POINT('Ctrl Pts',(-2.74486020807011,16.9,-1.07185368213596));
#456767=CARTESIAN_POINT('Ctrl Pts',(-2.75329837869529,16.9,-1.05430827125652));
#456768=CARTESIAN_POINT('Ctrl Pts',(-2.79594224914987,16.9,-0.965639262077881));
#456769=CARTESIAN_POINT('Ctrl Pts',(-2.83406860032868,16.9,-0.874811518173496));
#456770=CARTESIAN_POINT('Ctrl Pts',(-2.86771440442525,16.9,-0.782245644902387));
#456771=CARTESIAN_POINT('Ctrl Pts',(-2.89939603998739,16.9,-0.695083565076656));
#456772=CARTESIAN_POINT('Ctrl Pts',(-2.92710481817242,16.9,-0.606379438499839));
#456773=CARTESIAN_POINT('Ctrl Pts',(-2.95083879450907,16.9,-0.51645788495648));
#456774=CARTESIAN_POINT('Origin',(0.,16.9,0.));
#456775=CARTESIAN_POINT('Ctrl Pts',(2.5805589374942,6.77091034656191,-1.26059492705579));
#456776=CARTESIAN_POINT('Ctrl Pts',(2.16270489326978,6.82366602184023,-2.11598230427607));
#456777=CARTESIAN_POINT('Ctrl Pts',(0.416998689866887,6.92917737239689,
-3.36416092756532));
#456778=CARTESIAN_POINT('Ctrl Pts',(-2.59929056306034,7.08744439823184,
-2.18104546498594));
#456779=CARTESIAN_POINT('Ctrl Pts',(-3.24232899203514,7.24571142406682,
0.989791302620714));
#456780=CARTESIAN_POINT('Ctrl Pts',(-0.93866040260113,7.4039784499018,3.25840088127091));
#456781=CARTESIAN_POINT('Ctrl Pts',(2.22121069771714,7.56224547573676,2.5625637409689));
#456782=CARTESIAN_POINT('Ctrl Pts',(3.3586919237496,7.72051250157174,-0.465667476795367));
#456783=CARTESIAN_POINT('Ctrl Pts',(1.44022373180849,7.8787795274067,-3.06992192074064));
#456784=CARTESIAN_POINT('Ctrl Pts',(-1.78916098019484,8.03704655324167,
-2.88058449686228));
#456785=CARTESIAN_POINT('Ctrl Pts',(-3.39022251156056,8.19531357907665,
-0.0697920698937834));
#456786=CARTESIAN_POINT('Ctrl Pts',(-1.90617827987364,8.3535806049116,2.80448353848272));
#456787=CARTESIAN_POINT('Ctrl Pts',(1.31257158419998,8.5118476307466,3.12662922130667));
#456788=CARTESIAN_POINT('Ctrl Pts',(3.33683050597697,8.67011465658154,0.603461870573552));
#456789=CARTESIAN_POINT('Ctrl Pts',(2.32450679460257,8.82838168241653,-2.46886569239248));
#456790=CARTESIAN_POINT('Ctrl Pts',(-0.803177531322823,8.98664870825149,
-3.29447030739919));
#456791=CARTESIAN_POINT('Ctrl Pts',(-3.19994881461505,9.14491573408647,
-1.12202938400675));
#456792=CARTESIAN_POINT('Ctrl Pts',(-2.68469389625817,9.30318275992144,
2.07148374386093));
#456793=CARTESIAN_POINT('Ctrl Pts',(0.273695539681721,9.4614497857564,3.37989889026531));
#456794=CARTESIAN_POINT('Ctrl Pts',(2.98301528359298,9.61971681159137,1.61252745511383));
#456795=CARTESIAN_POINT('Ctrl Pts',(2.97772210058549,9.77798383742635,-1.62228130541839));
#456796=CARTESIAN_POINT('Ctrl Pts',(0.262632594907607,9.9362508632613,-3.3807764718047));
#456797=CARTESIAN_POINT('Ctrl Pts',(-2.69145861104891,10.0945178890963,
-2.06268657014607));
#456798=CARTESIAN_POINT('Ctrl Pts',(-3.19626004985765,10.2527849149312,
1.13249596744652));
#456799=CARTESIAN_POINT('Ctrl Pts',(-0.792390653220595,10.4110519407662,
3.29708089890013));
#456800=CARTESIAN_POINT('Ctrl Pts',(2.33257261886262,10.5693189666012,2.46124569460491));
#456801=CARTESIAN_POINT('Ctrl Pts',(3.33484068029608,10.7275859924362,-0.614380207850174));
#456802=CARTESIAN_POINT('Ctrl Pts',(1.30232632955009,10.8858530182711,-3.13090586417973));
#456803=CARTESIAN_POINT('Ctrl Pts',(-1.91533520282064,11.0441200441061,
-2.7982345253605));
#456804=CARTESIAN_POINT('Ctrl Pts',(-3.38999725238531,11.2023870699411,
0.0808951693976638));
#456805=CARTESIAN_POINT('Ctrl Pts',(-1.77968313098077,11.360654095776,2.88640838279897));
#456806=CARTESIAN_POINT('Ctrl Pts',(1.45018394022225,11.518921121611,3.06522298348167));
#456807=CARTESIAN_POINT('Ctrl Pts',(3.36034997176485,11.677188147446,0.454613535191446));
#456808=CARTESIAN_POINT('Ctrl Pts',(2.21251954598142,11.835455173281,-2.56970478025603));
#456809=CARTESIAN_POINT('Ctrl Pts',(-0.948755012143288,11.9937221991159,
-3.2555321110461));
#456810=CARTESIAN_POINT('Ctrl Pts',(-3.24664049163476,12.1519892249509,
-0.978749670253043));
#456811=CARTESIAN_POINT('Ctrl Pts',(-2.59000777962451,12.3102562507859,
2.18871768405023));
#456812=CARTESIAN_POINT('Ctrl Pts',(0.423592117726756,12.4685232766209,
3.36440115286681));
#456813=CARTESIAN_POINT('Ctrl Pts',(3.05171335757124,12.6267903024558,1.47840149529983));
#456814=CARTESIAN_POINT('Ctrl Pts',(2.90270462181359,12.7850573282908,-1.75297783143327));
#456815=CARTESIAN_POINT('Ctrl Pts',(0.112167317123486,12.9433243541258,
-3.38910665157133));
#456816=CARTESIAN_POINT('Ctrl Pts',(-2.78044484806947,13.1015913799607,
-1.94106976647485));
#456817=CARTESIAN_POINT('Ctrl Pts',(-3.14278767844486,13.2598584057957,
1.27338564834797));
#456818=CARTESIAN_POINT('Ctrl Pts',(-0.645120783207451,13.4181254316307,
3.32903057926365));
#456819=CARTESIAN_POINT('Ctrl Pts',(2.43962098791356,13.5763924574656,2.35518041283082));
#456820=CARTESIAN_POINT('Ctrl Pts',(3.30425105968087,13.7346594833006,-0.761938558424485));
#456821=CARTESIAN_POINT('Ctrl Pts',(1.16193595627524,13.8929265091356,-3.18567581146292));
#456822=CARTESIAN_POINT('Ctrl Pts',(-2.03776777487231,14.0511935349705,
-2.71037404638865));
#456823=CARTESIAN_POINT('Ctrl Pts',(-3.3830556511082,14.2094605608055,0.231430806858688));
#456824=CARTESIAN_POINT('Ctrl Pts',(-1.64968416256043,14.3677275866405,
2.96262862699381));
#456825=CARTESIAN_POINT('Ctrl Pts',(1.58493778894308,14.5259946124754,2.99776492739358));
#456826=CARTESIAN_POINT('Ctrl Pts',(3.37723035838085,14.6842616383104,0.304866953911748));
#456827=CARTESIAN_POINT('Ctrl Pts',(2.09616341132095,14.8425286641454,-2.66546967686099));
#456828=CARTESIAN_POINT('Ctrl Pts',(-1.09245796717358,15.0007956899804,
-3.21016193435995));
#456829=CARTESIAN_POINT('Ctrl Pts',(-3.28692286143165,15.1590627158153,
-0.833542173003866));
#456830=CARTESIAN_POINT('Ctrl Pts',(-2.49020085562839,15.3173297416503,
2.30163925299127));
#456831=CARTESIAN_POINT('Ctrl Pts',(0.572640891743325,15.4755967674853,
3.34223907283957));
#456832=CARTESIAN_POINT('Ctrl Pts',(3.11440623668499,15.6338637933202,1.34139399488469));
#456833=CARTESIAN_POINT('Ctrl Pts',(2.82191242834627,15.7921308191552,-1.88028594736362));
#456834=CARTESIAN_POINT('Ctrl Pts',(-0.0384385357557312,15.9503978449902,
-3.39060173370077));
#456835=CARTESIAN_POINT('Ctrl Pts',(-2.86409573659214,16.1086648708252,
-1.81589248079735));
#456836=CARTESIAN_POINT('Ctrl Pts',(-3.08280821480706,16.2669318966601,
1.4122865025187));
#456837=CARTESIAN_POINT('Ctrl Pts',(-0.497155858873794,16.4251989224951,
3.35338935516332));
#456838=CARTESIAN_POINT('Ctrl Pts',(2.54297493246889,16.58346594833,2.24645259117239));
#456839=CARTESIAN_POINT('Ctrl Pts',(3.26488853074936,16.741732974165,-0.912123640571359));
#456840=CARTESIAN_POINT('Ctrl Pts',(1.77123132985941,16.8472443247217,-2.45304161063505));
#456841=CARTESIAN_POINT('Ctrl Pts',(0.863261863496793,16.9,-2.73919020059434));
#456842=CARTESIAN_POINT('Ctrl Pts',(2.75127836581033,6.88060689770794,-1.34399083100445));
#456843=CARTESIAN_POINT('Ctrl Pts',(2.30578077409195,6.93336257298626,-2.25596720602134));
#456844=CARTESIAN_POINT('Ctrl Pts',(0.444585650547508,7.03887392354292,
-3.58672032040565));
#456845=CARTESIAN_POINT('Ctrl Pts',(-2.7712492005887,7.19714094937788,-2.32533468446622));
#456846=CARTESIAN_POINT('Ctrl Pts',(-3.45682847270599,7.35540797521285,
1.05527192500856));
#456847=CARTESIAN_POINT('Ctrl Pts',(-1.00075840973701,7.51367500104783,
3.47396361366696));
#456848=CARTESIAN_POINT('Ctrl Pts',(2.36815708788644,7.67194202688279,2.73209267926421));
#456849=CARTESIAN_POINT('Ctrl Pts',(3.58088950923443,7.83020905271776,-0.496474169201734));
#456850=CARTESIAN_POINT('Ctrl Pts',(1.53550315696296,7.98847607855273,-3.2730156411239));
#456851=CARTESIAN_POINT('Ctrl Pts',(-1.90752469406565,8.1467431043877,-3.07115241274106));
#456852=CARTESIAN_POINT('Ctrl Pts',(-3.6145060342613,8.30501013022267,-0.0744092332920613));
#456853=CARTESIAN_POINT('Ctrl Pts',(-2.03228338891822,8.46327715605764,
2.99001692020684));
#456854=CARTESIAN_POINT('Ctrl Pts',(1.39940605529955,8.62154418189262,3.33347446923435));
#456855=CARTESIAN_POINT('Ctrl Pts',(3.55758182775121,8.77981120772758,0.643384487359417));
#456856=CARTESIAN_POINT('Ctrl Pts',(2.4782868402065,8.93807823356255,-2.63219594363013));
#456857=CARTESIAN_POINT('Ctrl Pts',(-0.856312535135949,9.09634525939753,
-3.5124192483483));
#456858=CARTESIAN_POINT('Ctrl Pts',(-3.4116445927407,9.2546122852325,-1.19625834743339));
#456859=CARTESIAN_POINT('Ctrl Pts',(-2.86230247574601,9.41287931106746,
2.20852479933918));
#456860=CARTESIAN_POINT('Ctrl Pts',(0.29180213875536,9.57114633690244,3.60349944359066));
#456861=CARTESIAN_POINT('Ctrl Pts',(3.18035960945741,9.7294133627374,1.71920580346748));
#456862=CARTESIAN_POINT('Ctrl Pts',(3.17471625069386,9.88768038857238,-1.72960492938408));
#456863=CARTESIAN_POINT('Ctrl Pts',(0.280007313930059,10.0459474144073,
-3.60443508240459));
#456864=CARTESIAN_POINT('Ctrl Pts',(-2.86951471693306,10.2042144402423,
-2.19914563989808));
#456865=CARTESIAN_POINT('Ctrl Pts',(-3.40771179410311,10.3624814660773,
1.20741735805057));
#456866=CARTESIAN_POINT('Ctrl Pts',(-0.844812040446202,10.5207484919123,
3.51520254611148));
#456867=CARTESIAN_POINT('Ctrl Pts',(2.48688626704642,10.6790155177472,2.62407183735385));
#456868=CARTESIAN_POINT('Ctrl Pts',(3.55546036318475,10.8372825435822,-0.655025138035238));
#456869=CARTESIAN_POINT('Ctrl Pts',(1.38848301569722,10.9955495694172,-3.33803403764565));
#456870=CARTESIAN_POINT('Ctrl Pts',(-2.04204609715766,11.1538165952521,
-2.98335449744216));
#456871=CARTESIAN_POINT('Ctrl Pts',(-3.61426587284255,11.3120836210871,
0.0862468693229847));
#456872=CARTESIAN_POINT('Ctrl Pts',(-1.8974198283646,11.4703506469221,3.07736158361088));
#456873=CARTESIAN_POINT('Ctrl Pts',(1.54612229281355,11.628617672757,3.26800584102399));
#456874=CARTESIAN_POINT('Ctrl Pts',(3.5826572470557,11.786884698592,0.484688943160252));
#456875=CARTESIAN_POINT('Ctrl Pts',(2.35889096441335,11.945151724427,-2.73970614106683));
#456876=CARTESIAN_POINT('Ctrl Pts',(-1.01152083815554,12.1034187502619,
-3.47090505711113));
#456877=CARTESIAN_POINT('Ctrl Pts',(-3.46142520382508,12.2616857760969,
-1.04349982253303));
#456878=CARTESIAN_POINT('Ctrl Pts',(-2.76135230543533,12.4199528019319,
2.33351446676942));
#456879=CARTESIAN_POINT('Ctrl Pts',(0.451615273147389,12.5782198277669,
3.58697643804951));
#456880=CARTESIAN_POINT('Ctrl Pts',(3.25360247245234,12.7364868536018,1.57620660815046));
#456881=CARTESIAN_POINT('Ctrl Pts',(3.09473591643218,12.8947538794368,-1.86894781331778));
#456882=CARTESIAN_POINT('Ctrl Pts',(0.119587856905344,13.0530209052718,
-3.61331635345105));
#456883=CARTESIAN_POINT('Ctrl Pts',(-2.96438792645846,13.2112879311067,
-2.06948315631825));
#456884=CARTESIAN_POINT('Ctrl Pts',(-3.35070190508293,13.3695549569417,
1.35762773511193));
#456885=CARTESIAN_POINT('Ctrl Pts',(-0.68779938655336,13.5278219827767,
3.54926588917315));
#456886=CARTESIAN_POINT('Ctrl Pts',(2.60101652680755,13.6860890086117,2.5109897019805));
#456887=CARTESIAN_POINT('Ctrl Pts',(3.52284705596895,13.8443560344466,-0.812345357206038));
#456888=CARTESIAN_POINT('Ctrl Pts',(1.23880497845224,14.0026230602816,-3.39642734495106));
#456889=CARTESIAN_POINT('Ctrl Pts',(-2.17257831708182,14.1608900861166,
-2.88968152160239));
#456890=CARTESIAN_POINT('Ctrl Pts',(-3.6068650430687,14.3191571119515,0.246741340738604));
#456891=CARTESIAN_POINT('Ctrl Pts',(-1.7588206496379,14.4774241377865,3.15862425343142));
#456892=CARTESIAN_POINT('Ctrl Pts',(1.68979091564891,14.6356911636215,3.19608503052896));
#456893=CARTESIAN_POINT('Ctrl Pts',(3.60065437234059,14.7939581894564,0.325035728717899));
#456894=CARTESIAN_POINT('Ctrl Pts',(2.23483717460472,14.9522252152914,-2.84180645910457));
#456895=CARTESIAN_POINT('Ctrl Pts',(-1.16473060427767,15.1104922411264,
-3.42253337152165));
#456896=CARTESIAN_POINT('Ctrl Pts',(-3.50437249362942,15.2687592669614,
-0.888685979713743));
#456897=CARTESIAN_POINT('Ctrl Pts',(-2.65494255568738,15.4270262927963,
2.45390647376714));
#456898=CARTESIAN_POINT('Ctrl Pts',(0.610524516197086,15.5852933186313,
3.56334820370292));
#456899=CARTESIAN_POINT('Ctrl Pts',(3.32044286097821,15.7435603444663,1.4301352410644));
#456900=CARTESIAN_POINT('Ctrl Pts',(3.00859883551403,15.9018273703012,-2.00467812354714));
#456901=CARTESIAN_POINT('Ctrl Pts',(-0.040981475098891,16.0600943961362,
-3.61491034421719));
#456902=CARTESIAN_POINT('Ctrl Pts',(-3.05357282223019,16.2183614219712,
-1.9360246435242));
#456903=CARTESIAN_POINT('Ctrl Pts',(-3.28675444071701,16.3766284478061,
1.50571771264353));
#456904=CARTESIAN_POINT('Ctrl Pts',(-0.53004569633412,16.5348954736411,
3.57523614397983));
#456905=CARTESIAN_POINT('Ctrl Pts',(2.71120795376732,16.6931624994761,2.39506888376388));
#456906=CARTESIAN_POINT('Ctrl Pts',(3.48088046001204,16.8514295253111,-0.972466081974047));
#456907=CARTESIAN_POINT('Ctrl Pts',(1.88840888998243,16.9569408758677,-2.61532500409627));
#456908=CARTESIAN_POINT('Ctrl Pts',(0.92037180571978,17.009696551146,-2.92040403698463));
#456909=CARTESIAN_POINT('Ctrl Pts',(2.92199779412645,6.99030344885397,-1.42738673495312));
#456910=CARTESIAN_POINT('Ctrl Pts',(2.44885665491412,7.04305912413229,-2.39595210776662));
#456911=CARTESIAN_POINT('Ctrl Pts',(0.47217261122813,7.14857047468894,-3.80927971324597));
#456912=CARTESIAN_POINT('Ctrl Pts',(-2.94320783811705,7.3068375005239,-2.4696239039465));
#456913=CARTESIAN_POINT('Ctrl Pts',(-3.67132795337684,7.46510452635888,
1.12075254739641));
#456914=CARTESIAN_POINT('Ctrl Pts',(-1.06285641687289,7.62337155219385,
3.68952634606302));
#456915=CARTESIAN_POINT('Ctrl Pts',(2.51510347805574,7.78163857802882,2.90162161755951));
#456916=CARTESIAN_POINT('Ctrl Pts',(3.80308709471926,7.93990560386379,-0.5272808616081));
#456917=CARTESIAN_POINT('Ctrl Pts',(1.63078258211743,8.09817262969876,-3.47610936150716));
#456918=CARTESIAN_POINT('Ctrl Pts',(-2.02588840793647,8.25643965553374,
-3.26172032861983));
#456919=CARTESIAN_POINT('Ctrl Pts',(-3.83878955696203,8.41470668136869,
-0.07902639669034));
#456920=CARTESIAN_POINT('Ctrl Pts',(-2.15838849796279,8.57297370720367,
3.17555030193098));
#456921=CARTESIAN_POINT('Ctrl Pts',(1.48624052639912,8.73124073303864,3.54031971716202));
#456922=CARTESIAN_POINT('Ctrl Pts',(3.77833314952545,8.88950775887361,0.683307104145285));
#456923=CARTESIAN_POINT('Ctrl Pts',(2.63206688581044,9.04777478470857,-2.79552619486779));
#456924=CARTESIAN_POINT('Ctrl Pts',(-0.909447538949081,9.20604181054356,
-3.73036818929741));
#456925=CARTESIAN_POINT('Ctrl Pts',(-3.62334037086634,9.36430883637851,
-1.27048731086003));
#456926=CARTESIAN_POINT('Ctrl Pts',(-3.03991105523385,9.52257586221349,
2.34556585481744));
#456927=CARTESIAN_POINT('Ctrl Pts',(0.309908737829001,9.68084288804846,
3.82709999691602));
#456928=CARTESIAN_POINT('Ctrl Pts',(3.37770393532185,9.83910991388343,1.82588415182111));
#456929=CARTESIAN_POINT('Ctrl Pts',(3.37171040080224,9.9973769397184,-1.83692855334977));
#456930=CARTESIAN_POINT('Ctrl Pts',(0.297382032952511,10.1556439655534,
-3.82809369300449));
#456931=CARTESIAN_POINT('Ctrl Pts',(-3.04757082281721,10.3139109913884,
-2.33560470965009));
#456932=CARTESIAN_POINT('Ctrl Pts',(-3.61916353834856,10.4721780172233,
1.2823387486546));
#456933=CARTESIAN_POINT('Ctrl Pts',(-0.897233427671811,10.6304450430583,
3.73332419332284));
#456934=CARTESIAN_POINT('Ctrl Pts',(2.64119991523022,10.7887120688932,2.78689798010279));
#456935=CARTESIAN_POINT('Ctrl Pts',(3.77608004607342,10.9469790947282,-0.695670068220297));
#456936=CARTESIAN_POINT('Ctrl Pts',(1.47463970184435,11.1052461205632,-3.54516221111158));
#456937=CARTESIAN_POINT('Ctrl Pts',(-2.16875699149466,11.2635131463982,
-3.16847446952381));
#456938=CARTESIAN_POINT('Ctrl Pts',(-3.8385344932998,11.4217801722331,0.0915985692483058));
#456939=CARTESIAN_POINT('Ctrl Pts',(-2.01515652574843,11.5800471980681,
3.26831478442278));
#456940=CARTESIAN_POINT('Ctrl Pts',(1.64206064540484,11.7383142239031,3.47078869856631));
#456941=CARTESIAN_POINT('Ctrl Pts',(3.80496452234655,11.896581249738,0.514764351129056));
#456942=CARTESIAN_POINT('Ctrl Pts',(2.50526238284528,12.054848275573,-2.90970750187763));
#456943=CARTESIAN_POINT('Ctrl Pts',(-1.0742866641678,12.213115301408,-3.68627800317616));
#456944=CARTESIAN_POINT('Ctrl Pts',(-3.6762099160154,12.371382327243,-1.10824997481301));
#456945=CARTESIAN_POINT('Ctrl Pts',(-2.93269683124615,12.5296493530779,
2.47831124948861));
#456946=CARTESIAN_POINT('Ctrl Pts',(0.479638428568019,12.6879163789129,
3.8095517232322));
#456947=CARTESIAN_POINT('Ctrl Pts',(3.45549158733344,12.8461834047478,1.67401172100108));
#456948=CARTESIAN_POINT('Ctrl Pts',(3.28676721105077,13.0044504305828,-1.98491779520228));
#456949=CARTESIAN_POINT('Ctrl Pts',(0.127008396687204,13.1627174564178,
-3.83752605533076));
#456950=CARTESIAN_POINT('Ctrl Pts',(-3.14833100484746,13.3209844822528,
-2.19789654616165));
#456951=CARTESIAN_POINT('Ctrl Pts',(-3.55861613172099,13.4792515080877,
1.44186982187588));
#456952=CARTESIAN_POINT('Ctrl Pts',(-0.730477989899271,13.6375185339227,
3.76950119908265));
#456953=CARTESIAN_POINT('Ctrl Pts',(2.76241206570155,13.7957855597577,2.66679899113018));
#456954=CARTESIAN_POINT('Ctrl Pts',(3.74144305225704,13.9540525855927,-0.862752155987591));
#456955=CARTESIAN_POINT('Ctrl Pts',(1.31567400062923,14.1123196114276,-3.6071788784392));
#456956=CARTESIAN_POINT('Ctrl Pts',(-2.30738885929133,14.2705866372626,
-3.06898899681613));
#456957=CARTESIAN_POINT('Ctrl Pts',(-3.8306744350292,14.4288536630976,0.262051874618519));
#456958=CARTESIAN_POINT('Ctrl Pts',(-1.86795713671538,14.5871206889325,
3.35461987986903));
#456959=CARTESIAN_POINT('Ctrl Pts',(1.79464404235475,14.7453877147675,3.39440513366433));
#456960=CARTESIAN_POINT('Ctrl Pts',(3.82407838630033,14.9036547406025,0.345204503524049));
#456961=CARTESIAN_POINT('Ctrl Pts',(2.3735109378885,15.0619217664374,-3.01814324134815));
#456962=CARTESIAN_POINT('Ctrl Pts',(-1.23700324138176,15.2201887922724,
-3.63490480868335));
#456963=CARTESIAN_POINT('Ctrl Pts',(-3.72182212582719,15.3784558181074,
-0.943829786423622));
#456964=CARTESIAN_POINT('Ctrl Pts',(-2.81968425574637,15.5367228439423,
2.60617369454302));
#456965=CARTESIAN_POINT('Ctrl Pts',(0.648408140650847,15.6949898697773,
3.78445733456626));
#456966=CARTESIAN_POINT('Ctrl Pts',(3.52647948527143,15.8532568956123,1.51887648724411));
#456967=CARTESIAN_POINT('Ctrl Pts',(3.19528524268179,16.0115239214473,-2.12907029973066));
#456968=CARTESIAN_POINT('Ctrl Pts',(-0.0435244144420506,16.1697909472822,
-3.83921895473361));
#456969=CARTESIAN_POINT('Ctrl Pts',(-3.24304990786825,16.3280579731172,
-2.05615680625106));
#456970=CARTESIAN_POINT('Ctrl Pts',(-3.49070066662695,16.4863249989522,
1.59914892276836));
#456971=CARTESIAN_POINT('Ctrl Pts',(-0.562935533794447,16.6445920247871,
3.79708293279634));
#456972=CARTESIAN_POINT('Ctrl Pts',(2.87944097506574,16.8028590506221,2.54368517635538));
#456973=CARTESIAN_POINT('Ctrl Pts',(3.6968723892747,16.9611260764571,-1.03280852337674));
#456974=CARTESIAN_POINT('Ctrl Pts',(2.00558645010545,17.0666374270137,-2.7776083975575));
#456975=CARTESIAN_POINT('Ctrl Pts',(0.977481747942766,17.1193931022921,
-3.10161787337492));
#456976=CARTESIAN_POINT('Ctrl Pts',(3.09271722244258,7.1,-1.51078263890179));
#456977=CARTESIAN_POINT('Ctrl Pts',(2.5919325357363,7.15275567527832,-2.53593700951189));
#456978=CARTESIAN_POINT('Ctrl Pts',(0.49975957190875,7.25826702583497,-4.03183910608629));
#456979=CARTESIAN_POINT('Ctrl Pts',(-3.11516647564541,7.41653405166994,
-2.61391312342677));
#456980=CARTESIAN_POINT('Ctrl Pts',(-3.88582743404769,7.57480107750491,
1.18623316978426));
#456981=CARTESIAN_POINT('Ctrl Pts',(-1.12495442400877,7.73306810333987,
3.90508907845907));
#456982=CARTESIAN_POINT('Ctrl Pts',(2.66204986822505,7.89133512917485,3.07115055585482));
#456983=CARTESIAN_POINT('Ctrl Pts',(4.02528468020409,8.04960215500981,-0.558087554014467));
#456984=CARTESIAN_POINT('Ctrl Pts',(1.72606200727191,8.20786918084479,-3.67920308189041));
#456985=CARTESIAN_POINT('Ctrl Pts',(-2.14425212180729,8.36613620667976,
-3.45228824449861));
#456986=CARTESIAN_POINT('Ctrl Pts',(-4.06307307966276,8.52440323251473,
-0.0836435600886169));
#456987=CARTESIAN_POINT('Ctrl Pts',(-2.28449360700737,8.6826702583497,3.3610836836551));
#456988=CARTESIAN_POINT('Ctrl Pts',(1.5730749974987,8.84093728418467,3.7471649650897));
#456989=CARTESIAN_POINT('Ctrl Pts',(3.99908447129969,8.99920431001965,0.723229720931148));
#456990=CARTESIAN_POINT('Ctrl Pts',(2.78584693141438,9.1574713358546,-2.95885644610544));
#456991=CARTESIAN_POINT('Ctrl Pts',(-0.962582542762211,9.31573836168959,
-3.94831713024653));
#456992=CARTESIAN_POINT('Ctrl Pts',(-3.83503614899198,9.47400538752455,
-1.34471627428667));
#456993=CARTESIAN_POINT('Ctrl Pts',(-3.21751963472169,9.63227241335952,
2.48260691029569));
#456994=CARTESIAN_POINT('Ctrl Pts',(0.328015336902643,9.79053943919449,
4.05070055024137));
#456995=CARTESIAN_POINT('Ctrl Pts',(3.57504826118628,9.94880646502946,1.93256250017476));
#456996=CARTESIAN_POINT('Ctrl Pts',(3.56870455091062,10.1070734908644,-1.94425217731546));
#456997=CARTESIAN_POINT('Ctrl Pts',(0.31475675197496,10.2653405166994,-4.05175230360438));
#456998=CARTESIAN_POINT('Ctrl Pts',(-3.22562692870135,10.4236075425344,
-2.4720637794021));
#456999=CARTESIAN_POINT('Ctrl Pts',(-3.83061528259403,10.5818745683694,
1.35726013925865));
#457000=CARTESIAN_POINT('Ctrl Pts',(-0.949654814897419,10.7401415942043,
3.9514458405342));
#457001=CARTESIAN_POINT('Ctrl Pts',(2.79551356341402,10.8984086200393,2.94972412285173));
#457002=CARTESIAN_POINT('Ctrl Pts',(3.99669972896209,11.0566756458742,-0.736314998405361));
#457003=CARTESIAN_POINT('Ctrl Pts',(1.56079638799147,11.2149426717092,-3.7522903845775));
#457004=CARTESIAN_POINT('Ctrl Pts',(-2.29546788583168,11.3732096975442,
-3.35359444160547));
#457005=CARTESIAN_POINT('Ctrl Pts',(-4.06280311375705,11.5314767233792,
0.0969502691736263));
#457006=CARTESIAN_POINT('Ctrl Pts',(-2.13289322313227,11.6897437492141,
3.45926798523469));
#457007=CARTESIAN_POINT('Ctrl Pts',(1.73799899799614,11.8480107750491,3.67357155610862));
#457008=CARTESIAN_POINT('Ctrl Pts',(4.0272717976374,12.0062778008841,0.544839759097863));
#457009=CARTESIAN_POINT('Ctrl Pts',(2.6516338012772,12.164544826719,-3.07970886268844));
#457010=CARTESIAN_POINT('Ctrl Pts',(-1.13705249018005,12.322811852554,-3.90165094924119));
#457011=CARTESIAN_POINT('Ctrl Pts',(-3.89099462820572,12.481078878389,-1.17300012709299));
#457012=CARTESIAN_POINT('Ctrl Pts',(-3.10404135705697,12.6393459042239,
2.62310803220781));
#457013=CARTESIAN_POINT('Ctrl Pts',(0.507661583988647,12.7976129300589,
4.0321270084149));
#457014=CARTESIAN_POINT('Ctrl Pts',(3.65738070221454,12.9558799558939,1.77181683385171));
#457015=CARTESIAN_POINT('Ctrl Pts',(3.47879850566936,13.1141469817289,-2.10088777708678));
#457016=CARTESIAN_POINT('Ctrl Pts',(0.134428936469064,13.2724140075638,
-4.06173575721048));
#457017=CARTESIAN_POINT('Ctrl Pts',(-3.33227408323645,13.4306810333988,
-2.32630993600505));
#457018=CARTESIAN_POINT('Ctrl Pts',(-3.76653035835906,13.5889480592338,
1.52611190863984));
#457019=CARTESIAN_POINT('Ctrl Pts',(-0.77315659324518,13.7472150850688,
3.98973650899216));
#457020=CARTESIAN_POINT('Ctrl Pts',(2.92380760459554,13.9054821109037,2.82260828027986));
#457021=CARTESIAN_POINT('Ctrl Pts',(3.96003904854512,14.0637491367387,-0.913158954769142));
#457022=CARTESIAN_POINT('Ctrl Pts',(1.39254302280623,14.2220161625737,-3.81793041192735));
#457023=CARTESIAN_POINT('Ctrl Pts',(-2.44219940150084,14.3802831884086,
-3.24829647202987));
#457024=CARTESIAN_POINT('Ctrl Pts',(-4.0544838269897,14.5385502142436,0.277362408498434));
#457025=CARTESIAN_POINT('Ctrl Pts',(-1.97709362379286,14.6968172400786,
3.55061550630664));
#457026=CARTESIAN_POINT('Ctrl Pts',(1.89949716906058,14.8550842659136,3.59272523679971));
#457027=CARTESIAN_POINT('Ctrl Pts',(4.04750240026006,15.0133512917485,0.365373278330201));
#457028=CARTESIAN_POINT('Ctrl Pts',(2.51218470117228,15.1716183175835,-3.19448002359174));
#457029=CARTESIAN_POINT('Ctrl Pts',(-1.30927587848586,15.3298853434184,
-3.84727624584505));
#457030=CARTESIAN_POINT('Ctrl Pts',(-3.93927175802497,15.4881523692534,
-0.998973593133498));
#457031=CARTESIAN_POINT('Ctrl Pts',(-2.98442595580535,15.6464193950884,
2.7584409153189));
#457032=CARTESIAN_POINT('Ctrl Pts',(0.686291765104606,15.8046864209234,
4.0055664654296));
#457033=CARTESIAN_POINT('Ctrl Pts',(3.73251610956465,15.9629534467583,1.60761773342382));
#457034=CARTESIAN_POINT('Ctrl Pts',(3.38197164984955,16.1212204725933,-2.25346247591418));
#457035=CARTESIAN_POINT('Ctrl Pts',(-0.0460673537852081,16.2794874984283,
-4.06352756525002));
#457036=CARTESIAN_POINT('Ctrl Pts',(-3.4325269935063,16.4377545242632,-2.17628896897791));
#457037=CARTESIAN_POINT('Ctrl Pts',(-3.69464689253689,16.5960215500982,
1.6925801328932));
#457038=CARTESIAN_POINT('Ctrl Pts',(-0.595825371254773,16.7542885759332,
4.01892972161286));
#457039=CARTESIAN_POINT('Ctrl Pts',(3.04767399636416,16.9125556017682,2.69230146894688));
#457040=CARTESIAN_POINT('Ctrl Pts',(3.91286431853737,17.0708226276031,-1.09315096477943));
#457041=CARTESIAN_POINT('Ctrl Pts',(2.12276401022847,17.1763339781598,-2.93989179101872));
#457042=CARTESIAN_POINT('Ctrl Pts',(1.03459169016575,17.2290896534381,-3.28283170976521));
#457043=CARTESIAN_POINT('',(2.39254185396403,16.9,2.47449135723493));
#457044=CARTESIAN_POINT('Ctrl Pts',(2.39731517556588,16.9,2.47743591026517));
#457045=CARTESIAN_POINT('Ctrl Pts',(2.45735129193582,16.9,2.40997489184385));
#457046=CARTESIAN_POINT('Ctrl Pts',(2.51441069681728,16.9,2.34016593608869));
#457047=CARTESIAN_POINT('Ctrl Pts',(2.56829255542063,16.9,2.26807636518897));
#457048=CARTESIAN_POINT('Ctrl Pts',(2.63330364256217,16.9,2.18109678621307));
#457049=CARTESIAN_POINT('Ctrl Pts',(2.69369047677463,16.9,2.09079745741881));
#457050=CARTESIAN_POINT('Ctrl Pts',(2.74943143050006,16.9,1.99760261840811));
#457051=CARTESIAN_POINT('Ctrl Pts',(2.80611642770575,16.9,1.9028294070467));
#457052=CARTESIAN_POINT('Ctrl Pts',(2.85799705096988,16.9,1.80506084443894));
#457053=CARTESIAN_POINT('Ctrl Pts',(2.905000287014,16.9,1.70472487063112));
#457054=CARTESIAN_POINT('Ctrl Pts',(2.95127556121475,16.9,1.6059428485636));
#457055=CARTESIAN_POINT('Ctrl Pts',(2.99282330137881,16.9,1.50467138010401));
#457056=CARTESIAN_POINT('Ctrl Pts',(3.02952479600555,16.9,1.40131545622776));
#457057=CARTESIAN_POINT('Ctrl Pts',(3.03577281165996,16.9,1.38372027551583));
#457058=CARTESIAN_POINT('Ctrl Pts',(3.04188026153191,16.9,1.36606469584655));
#457059=CARTESIAN_POINT('Ctrl Pts',(3.04784641699272,16.9,1.34835073551));
#457060=CARTESIAN_POINT('Ctrl Pts',(3.05280703409911,16.9,1.33362229351004));
#457061=CARTESIAN_POINT('Ctrl Pts',(3.05766701641074,16.9,1.3188622323021));
#457062=CARTESIAN_POINT('Ctrl Pts',(3.062425668889,16.9,1.30407382307151));
#457063=CARTESIAN_POINT('Ctrl Pts',(3.09578122089829,16.9,1.20041516014575));
#457064=CARTESIAN_POINT('Ctrl Pts',(3.12417343625608,16.9,1.09533201835296));
#457065=CARTESIAN_POINT('Ctrl Pts',(3.1475702326327,16.9,0.989239984693864));
#457066=CARTESIAN_POINT('Ctrl Pts',(3.17093000708061,16.9,0.88331582580031));
#457067=CARTESIAN_POINT('Ctrl Pts',(3.18931018407837,16.9,0.776384998044518));
#457068=CARTESIAN_POINT('Ctrl Pts',(3.20262740083768,16.9,0.668856247340615));
#457069=CARTESIAN_POINT('Ctrl Pts',(3.21574256775655,16.9,0.562958931140931));
#457070=CARTESIAN_POINT('Ctrl Pts',(3.22394715946814,16.9,0.456480829259066));
#457071=CARTESIAN_POINT('Ctrl Pts',(3.22711221816567,16.9,0.349821217468776));
#457072=CARTESIAN_POINT('Ctrl Pts',(3.22862484445679,16.9,0.298847081311038));
#457073=CARTESIAN_POINT('Ctrl Pts',(3.22898570853728,16.9,0.247831699353688));
#457074=CARTESIAN_POINT('Ctrl Pts',(3.22817673574291,16.9,0.196820252878376));
#457075=CARTESIAN_POINT('Ctrl Pts',(3.22763618635905,16.9,0.162734797651577));
#457076=CARTESIAN_POINT('Ctrl Pts',(3.22657327371452,16.9,0.128651123411333));
#457077=CARTESIAN_POINT('Ctrl Pts',(3.22498195597518,16.9,0.094583064930471));
#457078=CARTESIAN_POINT('Ctrl Pts',(3.22426784467463,16.9,0.0792948638707587));
#457079=CARTESIAN_POINT('Ctrl Pts',(3.22344752043097,16.9,0.0640149857196622));
#457080=CARTESIAN_POINT('Ctrl Pts',(3.22252120818967,16.9,0.0487525626872403));
#457081=CARTESIAN_POINT('Ctrl Pts',(3.21617357369505,16.9,-0.0558345069773061));
#457082=CARTESIAN_POINT('Ctrl Pts',(3.20484788704636,16.9,-0.159716937956681));
#457083=CARTESIAN_POINT('Ctrl Pts',(3.18847069149561,16.9,-0.262520661788208));
#457084=CARTESIAN_POINT('Ctrl Pts',(3.17254566312765,16.9,-0.362486019915367));
#457085=CARTESIAN_POINT('Ctrl Pts',(3.15184400884743,16.9,-0.461432124162015));
#457086=CARTESIAN_POINT('Ctrl Pts',(3.12625233656091,16.9,-0.559000390964261));
#457087=CARTESIAN_POINT('Ctrl Pts',(3.10090297957557,16.9,-0.655644830527274));
#457088=CARTESIAN_POINT('Ctrl Pts',(3.07075571579294,16.9,-0.750938069922472));
#457089=CARTESIAN_POINT('Ctrl Pts',(3.03565640665044,16.9,-0.844506858436016));
#457090=CARTESIAN_POINT('Ctrl Pts',(3.01435271014496,16.9,-0.901298890005243));
#457091=CARTESIAN_POINT('Ctrl Pts',(2.99122368350055,16.9,-0.957455063351064));
#457092=CARTESIAN_POINT('Ctrl Pts',(2.96632347592632,16.9,-1.01291655518183));
#457093=CARTESIAN_POINT('Ctrl Pts',(2.95748571229695,16.9,-1.03260135314472));
#457094=CARTESIAN_POINT('Ctrl Pts',(2.94842479238806,16.9,-1.05219859840326));
#457095=CARTESIAN_POINT('Ctrl Pts',(2.93914302970222,16.9,-1.07170551931792));
#457096=CARTESIAN_POINT('Ctrl Pts',(2.9310199030181,16.9,-1.0887774048175));
#457097=CARTESIAN_POINT('Ctrl Pts',(2.92272610853918,16.9,-1.10578292304522));
#457098=CARTESIAN_POINT('Ctrl Pts',(2.91427468627422,16.9,-1.12269777829202));
#457099=CARTESIAN_POINT('Ctrl Pts',(2.86885951147453,16.9,-1.21359266954957));
#457100=CARTESIAN_POINT('Ctrl Pts',(2.81883571822984,16.9,-1.30200379923635));
#457101=CARTESIAN_POINT('Ctrl Pts',(2.76453606118357,16.9,-1.38770856780535));
#457102=CARTESIAN_POINT('Ctrl Pts',(2.70969650094221,16.9,-1.47426550157946));
#457103=CARTESIAN_POINT('Ctrl Pts',(2.65049488456746,16.9,-1.55806261189768));
#457104=CARTESIAN_POINT('Ctrl Pts',(2.58723209997326,16.9,-1.638836948331));
#457105=CARTESIAN_POINT('Ctrl Pts',(2.5244237260005,16.9,-1.71903109031586));
#457106=CARTESIAN_POINT('Ctrl Pts',(2.45761150944921,16.9,-1.79624623243237));
#457107=CARTESIAN_POINT('Ctrl Pts',(2.38706056192649,16.9,-1.87018374462621));
#457108=CARTESIAN_POINT('Ctrl Pts',(2.33201555442374,16.9,-1.92787100548312));
#457109=CARTESIAN_POINT('Ctrl Pts',(2.27469394955488,16.9,-1.98356231505416));
#457110=CARTESIAN_POINT('Ctrl Pts',(2.21521378714993,16.9,-2.03709518630478));
#457111=CARTESIAN_POINT('Ctrl Pts',(2.17274572791687,16.9,-2.07531695731658));
#457112=CARTESIAN_POINT('Ctrl Pts',(2.1292737737331,16.9000000000006,-2.1123511370141));
#457113=CARTESIAN_POINT('Ctrl Pts',(2.08484969764403,16.9000000000009,-2.14815125844571));
#457114=CARTESIAN_POINT('Ctrl Pts',(-0.000213030569266609,16.2776795453431,
-3.44751024702897));
#457115=CARTESIAN_POINT('Ctrl Pts',(-0.0131882280058195,16.2782821963715,
-3.4475237333034));
#457116=CARTESIAN_POINT('Ctrl Pts',(-0.0261632960604996,16.2788848473999,
-3.44745721540563));
#457117=CARTESIAN_POINT('Ctrl Pts',(-0.0391374597995815,16.2794874984283,
-3.44731028431536));
#457118=CARTESIAN_POINT('Ctrl Pts',(-1.17488723369223,16.3322431737066,
-3.43444803315932));
#457119=CARTESIAN_POINT('Ctrl Pts',(-2.30370711359927,16.3849988489849,
-2.80536850106861));
#457120=CARTESIAN_POINT('Ctrl Pts',(-2.91180370339122,16.4377545242632,
-1.84601721804475));
#457121=CARTESIAN_POINT('Ctrl Pts',(-3.51990029318317,16.4905101995416,
-0.886665935020874));
#457122=CARTESIAN_POINT('Ctrl Pts',(-3.60727359286003,16.5432658748199,
0.402957098936157));
#457123=CARTESIAN_POINT('Ctrl Pts',(-3.13448998915144,16.5960215500982,
1.43549354736796));
#457124=CARTESIAN_POINT('Ctrl Pts',(-2.66170638544285,16.6487772253765,
2.46802999579975));
#457125=CARTESIAN_POINT('Ctrl Pts',(-1.62876587834881,16.7015329006548,
3.2434798587063));
#457126=CARTESIAN_POINT('Ctrl Pts',(-0.505045730198636,16.7542885759332,
3.41010008138192));
#457127=CARTESIAN_POINT('Ctrl Pts',(0.52952772043461,16.8028590506221,3.56350202847929));
#457128=CARTESIAN_POINT('Ctrl Pts',(1.64104871889364,16.8514295253111,3.20084170308472));
#457129=CARTESIAN_POINT('Ctrl Pts',(2.39731517556588,16.9,2.47743591026517));
#457130=CARTESIAN_POINT('',(-2.33836210323076,7.1,-1.66746714335672));
#457131=CARTESIAN_POINT('Ctrl Pts',(-2.34138343307718,7.1,-1.67104082391619));
#457132=CARTESIAN_POINT('Ctrl Pts',(-2.30373709690902,7.1,-1.73710495792299));
#457133=CARTESIAN_POINT('Ctrl Pts',(-2.26340583681328,7.1,-1.8014079853077));
#457134=CARTESIAN_POINT('Ctrl Pts',(-2.22043566451384,7.1,-1.86376505338026));
#457135=CARTESIAN_POINT('Ctrl Pts',(-2.16722286282088,7.1,-1.94098592823214));
#457136=CARTESIAN_POINT('Ctrl Pts',(-2.10996506901757,7.1,-2.01522395346306));
#457137=CARTESIAN_POINT('Ctrl Pts',(-2.04905120510384,7.1,-2.08640434099551));
#457138=CARTESIAN_POINT('Ctrl Pts',(-1.98660349854121,7.1,-2.15937708756));
#457139=CARTESIAN_POINT('Ctrl Pts',(-1.92031284996429,7.1,-2.22913678539083));
#457140=CARTESIAN_POINT('Ctrl Pts',(-1.85054859855047,7.1,-2.29557990141108));
#457141=CARTESIAN_POINT('Ctrl Pts',(-1.77672045443771,7.1,-2.36589344804037));
#457142=CARTESIAN_POINT('Ctrl Pts',(-1.69900186632332,7.1,-2.4324936506496));
#457143=CARTESIAN_POINT('Ctrl Pts',(-1.61778142754668,7.1,-2.49522128635037));
#457144=CARTESIAN_POINT('Ctrl Pts',(-1.60259405024534,7.1,-2.50695070181474));
#457145=CARTESIAN_POINT('Ctrl Pts',(-1.58728087558103,7.1,-2.51854687198231));
#457146=CARTESIAN_POINT('Ctrl Pts',(-1.57186648200357,7.1,-2.52999246926519));
#457147=CARTESIAN_POINT('Ctrl Pts',(-1.49169164059863,7.1,-2.58952442180871));
#457148=CARTESIAN_POINT('Ctrl Pts',(-1.40867503025123,7.1,-2.64507039187443));
#457149=CARTESIAN_POINT('Ctrl Pts',(-1.32323616805416,7.1,-2.69654192373782));
#457150=CARTESIAN_POINT('Ctrl Pts',(-1.23618678154192,7.1,-2.74898369503879));
#457151=CARTESIAN_POINT('Ctrl Pts',(-1.14662232673984,7.1,-2.79719654281982));
#457152=CARTESIAN_POINT('Ctrl Pts',(-1.05494136675663,7.1,-2.8410556336148));
#457153=CARTESIAN_POINT('Ctrl Pts',(-0.962668701398649,7.1,-2.88519778928781));
#457154=CARTESIAN_POINT('Ctrl Pts',(-0.868251334078741,7.1,-2.92493036313033));
#457155=CARTESIAN_POINT('Ctrl Pts',(-0.772061266501809,7.1,-2.96008626738923));
#457156=CARTESIAN_POINT('Ctrl Pts',(-0.725618951099568,7.1,-2.9770601778456));
#457157=CARTESIAN_POINT('Ctrl Pts',(-0.678762960049247,7.1,-2.99296656202763));
#457158=CARTESIAN_POINT('Ctrl Pts',(-0.631533175966222,7.1,-3.00778272556646));
#457159=CARTESIAN_POINT('Ctrl Pts',(-0.610048859625699,7.1,-3.01452243760625));
#457160=CARTESIAN_POINT('Ctrl Pts',(-0.588487182318978,7.1,-3.02103651981684));
#457161=CARTESIAN_POINT('Ctrl Pts',(-0.566851836242806,7.1,-3.02732264566703));
#457162=CARTESIAN_POINT('Ctrl Pts',(-0.549634368029798,7.1,-3.03232516199506));
#457163=CARTESIAN_POINT('Ctrl Pts',(-0.532368322853267,7.1,-3.03718373790698));
#457164=CARTESIAN_POINT('Ctrl Pts',(-0.515077130872961,7.1,-3.04189155649519));
#457165=CARTESIAN_POINT('Ctrl Pts',(-0.413793396541499,7.1,-3.06946776105711));
#457166=CARTESIAN_POINT('Ctrl Pts',(-0.311489387944635,7.1,-3.09192266352597));
#457167=CARTESIAN_POINT('Ctrl Pts',(-0.208582244309945,7.1,-3.10913113842233));
#457168=CARTESIAN_POINT('Ctrl Pts',(-0.106239991649575,7.1,-3.12624515037076));
#457169=CARTESIAN_POINT('Ctrl Pts',(-0.00330032138165767,7.1,-3.13817062977676));
#457170=CARTESIAN_POINT('Ctrl Pts',(0.0998536181159393,7.1,-3.14474156889126));
#457171=CARTESIAN_POINT('Ctrl Pts',(0.195429067372106,7.1,-3.15082975574056));
#457172=CARTESIAN_POINT('Ctrl Pts',(0.29118926919932,7.1,-3.15232115511315));
#457173=CARTESIAN_POINT('Ctrl Pts',(0.386840550730246,7.1,-3.14904531704776));
#457174=CARTESIAN_POINT('Ctrl Pts',(0.454955630096398,7.1,-3.14671253105427));
#457175=CARTESIAN_POINT('Ctrl Pts',(0.523015704606009,7.1,-3.1419613991929));
#457176=CARTESIAN_POINT('Ctrl Pts',(0.590937668894151,7.1,-3.13485612111357));
#457177=CARTESIAN_POINT('Ctrl Pts',(0.610040322753848,7.1,-3.13285780335069));
#457178=CARTESIAN_POINT('Ctrl Pts',(0.629132049928093,7.1,-3.1306732129464));
#457179=CARTESIAN_POINT('Ctrl Pts',(0.648210991323371,7.1,-3.12830363025409));
#457180=CARTESIAN_POINT('Ctrl Pts',(0.662368701450295,7.1,-3.12654525885472));
#457181=CARTESIAN_POINT('Ctrl Pts',(0.67651570470214,7.1,-3.12468543554251));
#457182=CARTESIAN_POINT('Ctrl Pts',(0.690643043116382,7.1,-3.12272607557076));
#457183=CARTESIAN_POINT('Ctrl Pts',(0.791166298898776,7.1,-3.10878422482474));
#457184=CARTESIAN_POINT('Ctrl Pts',(0.890816293294953,7.1,-3.08979193939395));
#457185=CARTESIAN_POINT('Ctrl Pts',(0.989319276565167,7.1,-3.06604774520952));
#457186=CARTESIAN_POINT('Ctrl Pts',(1.09029556873711,7.1,-3.04170735865719));
#457187=CARTESIAN_POINT('Ctrl Pts',(1.19006716835258,7.1,-3.01237334165454));
#457188=CARTESIAN_POINT('Ctrl Pts',(1.28834555064191,7.1,-2.97831324493603));
#457189=CARTESIAN_POINT('Ctrl Pts',(1.38872832987599,7.1,-2.94352383255519));
#457190=CARTESIAN_POINT('Ctrl Pts',(1.48755403371945,7.1,-2.90380361678363));
#457191=CARTESIAN_POINT('Ctrl Pts',(1.58451087530088,7.1,-2.85938404168432));
#457192=CARTESIAN_POINT('Ctrl Pts',(1.66204961236623,7.1,-2.8238606304634));
#457193=CARTESIAN_POINT('Ctrl Pts',(1.73839317987524,7.1,-2.7853305896715));
#457194=CARTESIAN_POINT('Ctrl Pts',(1.81337498090191,7.1,-2.74388965300041));
#457195=CARTESIAN_POINT('Ctrl Pts',(1.83201173369785,7.1,-2.73358949373781));
#457196=CARTESIAN_POINT('Ctrl Pts',(1.85056706527456,7.1,-2.72310771383178));
#457197=CARTESIAN_POINT('Ctrl Pts',(1.86901608090916,7.1,-2.71245879056604));
#457198=CARTESIAN_POINT('Ctrl Pts',(1.96370706453454,7.1,-2.65780237753265));
#457199=CARTESIAN_POINT('Ctrl Pts',(2.05571727561232,7.1,-2.59868305315288));
#457200=CARTESIAN_POINT('Ctrl Pts',(2.14472625872352,7.1,-2.53537052888058));
#457201=CARTESIAN_POINT('Ctrl Pts',(2.23431822939319,7.1,-2.47164332271151));
#457202=CARTESIAN_POINT('Ctrl Pts',(2.32087037637371,7.1,-2.40366745534427));
#457203=CARTESIAN_POINT('Ctrl Pts',(2.40403967322767,7.1,-2.33166808527891));
#457204=CARTESIAN_POINT('Ctrl Pts',(2.44227422344943,7.1,-2.29856856857224));
#457205=CARTESIAN_POINT('Ctrl Pts',(2.47979353198495,7.1,-2.264618059125));
#457206=CARTESIAN_POINT('Ctrl Pts',(2.51656236325742,7.1,-2.22983524836611));
#457207=CARTESIAN_POINT('Ctrl Pts',(2.53389141267929,7.1,-2.21344220497005));
#457208=CARTESIAN_POINT('Ctrl Pts',(2.55105569210745,7.1,-2.19686218293923));
#457209=CARTESIAN_POINT('Ctrl Pts',(2.56803402823707,7.1,-2.1801146041988));
#457210=CARTESIAN_POINT('Ctrl Pts',(2.64761340219944,7.1,-2.10161681611318));
#457211=CARTESIAN_POINT('Ctrl Pts',(2.72319134043281,7.1,-2.01936632456138));
#457212=CARTESIAN_POINT('Ctrl Pts',(2.7944263119065,7.1,-1.93361058917696));
#457213=CARTESIAN_POINT('Ctrl Pts',(2.86463899052335,7.1,-1.84908553408765));
#457214=CARTESIAN_POINT('Ctrl Pts',(2.93063320931567,7.1,-1.76115460554111));
#457215=CARTESIAN_POINT('Ctrl Pts',(2.99205373512871,7.1,-1.67001353083844));
#457216=CARTESIAN_POINT('Ctrl Pts',(3.02712386093307,7.1,-1.61797345281149));
#457217=CARTESIAN_POINT('Ctrl Pts',(3.06070228237189,7.1,-1.56488607880856));
#457218=CARTESIAN_POINT('Ctrl Pts',(3.09271722244258,7.1,-1.51078263890179));
#457219=CARTESIAN_POINT('Ctrl Pts',(-2.34138343307717,7.1,-1.67104082391619));
#457220=CARTESIAN_POINT('Ctrl Pts',(-2.84455475580173,7.14857047468894,
-0.957347532745108));
#457221=CARTESIAN_POINT('Ctrl Pts',(-3.18141096386486,7.24989662465621,
1.04978223311021));
#457222=CARTESIAN_POINT('Ctrl Pts',(-0.93866040260113,7.4039784499018,3.25840088127091));
#457223=CARTESIAN_POINT('Ctrl Pts',(2.22121069771714,7.56224547573676,2.5625637409689));
#457224=CARTESIAN_POINT('Ctrl Pts',(3.3586919237496,7.72051250157174,-0.465667476795367));
#457225=CARTESIAN_POINT('Ctrl Pts',(1.7976392878798,7.84929397362782,-2.58474262293216));
#457226=CARTESIAN_POINT('Ctrl Pts',(0.422335728259563,7.92531977040558,
-2.86880237445628));
#457227=CARTESIAN_POINT('Ctrl Pts',(0.000911915543898995,7.94858989190502,
-2.86762206492074));
#457228=CARTESIAN_POINT('Origin',(0.,5.25141010809499,0.));
#457229=CARTESIAN_POINT('',(-2.33836210323078,7.1,1.66746714335669));
#457230=CARTESIAN_POINT('Origin',(0.,7.1,0.));
#457231=CARTESIAN_POINT('Ctrl Pts',(-2.33836210323078,7.1,1.66746714335669));
#457232=CARTESIAN_POINT('Ctrl Pts',(-1.78564062664172,7.15275567527832,
2.44257264372404));
#457233=CARTESIAN_POINT('Ctrl Pts',(0.141420484832718,7.25826702583498,
3.38695776202909));
#457234=CARTESIAN_POINT('Ctrl Pts',(2.92232820013613,7.41653405166992,1.72431918607449));
#457235=CARTESIAN_POINT('Ctrl Pts',(3.03563126175005,7.57480107750492,-1.50907675260125));
#457236=CARTESIAN_POINT('Ctrl Pts',(1.1700442784882,7.68642642964658,-2.82041444291808));
#457237=CARTESIAN_POINT('Ctrl Pts',(0.111967252847952,7.74529610650994,
-2.87593112245951));
#457238=CARTESIAN_POINT('Ctrl Pts',(0.00198847260380112,7.75141010809497,
-2.87512062938712));
#457239=CARTESIAN_POINT('Ctrl Pts',(-2.80245207497228,6.77091034656191,
1.99840595662732));
#457240=CARTESIAN_POINT('Ctrl Pts',(-2.14003309084293,6.82366602184023,
2.92734506953276));
#457241=CARTESIAN_POINT('Ctrl Pts',(0.169487920889316,6.92917737239688,
4.05916038193041));
#457242=CARTESIAN_POINT('Ctrl Pts',(3.50231673567846,7.08744439823185,2.06654130865895));
#457243=CARTESIAN_POINT('Ctrl Pts',(3.63810682553751,7.24571142406682,-1.8085801470938));
#457244=CARTESIAN_POINT('Ctrl Pts',(0.468031859858225,7.40397844990178,
-4.03685404743849));
#457245=CARTESIAN_POINT('Ctrl Pts',(-3.13048342197373,7.56224547573677,
-2.59201645208381));
#457246=CARTESIAN_POINT('Ctrl Pts',(-3.87887915070217,7.72051250157172,
1.21188621595859));
#457247=CARTESIAN_POINT('Ctrl Pts',(-1.09808361260071,7.87877952740671,
3.91280404022221));
#457248=CARTESIAN_POINT('Ctrl Pts',(2.68234612450716,8.03704655324167,3.0530522589568));
#457249=CARTESIAN_POINT('Ctrl Pts',(4.02159543523717,8.19531357907664,-0.58508579160953));
#457250=CARTESIAN_POINT('Ctrl Pts',(1.70119475466967,8.35358060491161,-3.69076252266703));
#457251=CARTESIAN_POINT('Ctrl Pts',(-2.16738208411717,8.51184763074659,
-3.43776992741298));
#457252=CARTESIAN_POINT('Ctrl Pts',(-4.06356523557141,8.67011465658154,
-0.0563216087165039));
#457253=CARTESIAN_POINT('Ctrl Pts',(-2.26182306892026,8.82838168241653,
3.37637792223869));
#457254=CARTESIAN_POINT('Ctrl Pts',(1.59823751538639,8.98664870825149,3.73649662230098));
#457255=CARTESIAN_POINT('Ctrl Pts',(4.00386126750968,9.14491573408645,0.696315939262238));
#457256=CARTESIAN_POINT('Ctrl Pts',(2.76588022140732,9.30318275992145,-2.97752802088584));
#457257=CARTESIAN_POINT('Ctrl Pts',(-0.989116986028071,9.46144978575638,
-3.94175258412388));
#457258=CARTESIAN_POINT('Ctrl Pts',(-3.84399427661538,9.61971681159139,
-1.3188907158956));
#457259=CARTESIAN_POINT('Ctrl Pts',(-3.20074783119648,9.77798383742633,
2.50419225677886));
#457260=CARTESIAN_POINT('Ctrl Pts',(0.355253556140568,9.93625086326132,
4.04840218967418));
#457261=CARTESIAN_POINT('Ctrl Pts',(3.58796589222327,10.0945178890963,1.90847216484256));
#457262=CARTESIAN_POINT('Ctrl Pts',(3.55554603797885,10.2527849149312,-1.9682118119268));
#457263=CARTESIAN_POINT('Ctrl Pts',(0.287496757183279,10.4110519407662,
-4.05377736788959));
#457264=CARTESIAN_POINT('Ctrl Pts',(-3.24218123459167,10.5693189666012,
-2.45031144180059));
#457265=CARTESIAN_POINT('Ctrl Pts',(-3.82139906738593,10.7275859924362,
1.38299475915826));
#457266=CARTESIAN_POINT('Ctrl Pts',(-0.923055063715857,10.8858530182711,
3.95774363494844));
#457267=CARTESIAN_POINT('Ctrl Pts',(2.8152904677005,11.0441200441061,2.9308539560656));
#457268=CARTESIAN_POINT('Ctrl Pts',(3.99165634033771,11.2023870699411,-0.763180838442537));
#457269=CARTESIAN_POINT('Ctrl Pts',(1.53552230930483,11.3606540957761,-3.7627033590557));
#457270=CARTESIAN_POINT('Ctrl Pts',(-2.3179726575683,11.518921121611,-3.33807850257005));
#457271=CARTESIAN_POINT('Ctrl Pts',(-4.06205871341305,11.677188147446,0.124275257374031));
#457272=CARTESIAN_POINT('Ctrl Pts',(-2.10957707260641,11.835455173281,3.47353564907578));
#457273=CARTESIAN_POINT('Ctrl Pts',(1.76266866080478,11.9937221991159,3.6617979904723));
#457274=CARTESIAN_POINT('Ctrl Pts',(4.03084500695705,12.1519892249509,0.51773918187053));
#457275=CARTESIAN_POINT('Ctrl Pts',(2.63085885380488,12.3102562507859,-3.09747429722644));
#457276=CARTESIAN_POINT('Ctrl Pts',(-1.16326991025864,12.4685232766208,
-3.89391428352127));
#457277=CARTESIAN_POINT('Ctrl Pts',(-3.89879605996908,12.6267903024558,
-1.14680190620711));
#457278=CARTESIAN_POINT('Ctrl Pts',(-3.08632731697582,12.7850573282908,
2.64392681878965));
#457279=CARTESIAN_POINT('Ctrl Pts',(0.534770909157417,12.9433243541257,
4.02862078269923));
#457280=CARTESIAN_POINT('Ctrl Pts',(3.66921519590491,13.1015913799607,1.74717634081329));
#457281=CARTESIAN_POINT('Ctrl Pts',(3.46458850694724,13.2598584057957,-2.1242391135025));
#457282=CARTESIAN_POINT('Ctrl Pts',(0.107105868234875,13.4181254316307,
-4.06254768560135));
#457283=CARTESIAN_POINT('Ctrl Pts',(-3.34784558382811,13.5763924574656,
-2.30384356990207));
#457284=CARTESIAN_POINT('Ctrl Pts',(-3.75617988553842,13.7346594833006,
1.55141163009235));
#457285=CARTESIAN_POINT('Ctrl Pts',(-0.746303276805527,13.8929265091356,
3.99484629952762));
#457286=CARTESIAN_POINT('Ctrl Pts',(2.94272654522848,14.0511935349705,2.8028780207378));
#457287=CARTESIAN_POINT('Ctrl Pts',(3.95380708902251,14.2094605608055,-0.939774094818543));
#457288=CARTESIAN_POINT('Ctrl Pts',(1.36683110091601,14.3677275866405,-3.82721037518206));
#457289=CARTESIAN_POINT('Ctrl Pts',(-2.46399228198733,14.5259946124754,
-3.23179562643458));
#457290=CARTESIAN_POINT('Ctrl Pts',(-4.05252671336466,14.6842616383104,
0.304626659242042));
#457291=CARTESIAN_POINT('Ctrl Pts',(-1.95316546723355,14.8425286641454,
3.56383446956885));
#457292=CARTESIAN_POINT('Ctrl Pts',(1.9236172112469,15.0007956899804,3.57986471419629));
#457293=CARTESIAN_POINT('Ctrl Pts',(4.04987218927447,15.1590627158153,0.338145564688239));
#457294=CARTESIAN_POINT('Ctrl Pts',(2.49063293224919,15.3173297416503,-3.2113142463538));
#457295=CARTESIAN_POINT('Ctrl Pts',(-1.33510822231294,15.4755967674853,
-3.83836439945144));
#457296=CARTESIAN_POINT('Ctrl Pts',(-3.94593125363753,15.6338637933202,
-0.972489264283366));
#457297=CARTESIAN_POINT('Ctrl Pts',(-2.96574720213873,15.7921308191552,
2.77851877993432));
#457298=CARTESIAN_POINT('Ctrl Pts',(0.713108371959378,15.9503978449902,
4.00073094771741));
#457299=CARTESIAN_POINT('Ctrl Pts',(3.74345621443102,16.1086648708251,1.58272275328413));
#457300=CARTESIAN_POINT('Ctrl Pts',(3.36632985623942,16.2669318966601,-2.27663517524305));
#457301=CARTESIAN_POINT('Ctrl Pts',(-0.0726117846316149,16.4251989224951,
-4.06220518329848));
#457302=CARTESIAN_POINT('Ctrl Pts',(-3.44861801907735,16.58346594833,-2.15495922372147));
#457303=CARTESIAN_POINT('Ctrl Pts',(-3.68007291451166,16.741732974165,1.72121251024924));
#457304=CARTESIAN_POINT('Ctrl Pts',(-1.61086821599449,16.8472443247217,
3.24872196051297));
#457305=CARTESIAN_POINT('Ctrl Pts',(-0.481137492902315,16.9,3.40820637768954));
#457306=CARTESIAN_POINT('Ctrl Pts',(-2.64775541772511,6.88060689770794,
1.88809301887045));
#457307=CARTESIAN_POINT('Ctrl Pts',(-2.02190226944253,6.93336257298626,
2.76575426092985));
#457308=CARTESIAN_POINT('Ctrl Pts',(0.160132108870451,7.03887392354293,
3.8350928419633));
#457309=CARTESIAN_POINT('Ctrl Pts',(3.30898722383101,7.19714094937786,1.95246726779747));
#457310=CARTESIAN_POINT('Ctrl Pts',(3.43728163760836,7.35540797521287,-1.70874568226295));
#457311=CARTESIAN_POINT('Ctrl Pts',(0.442196283631292,7.51367500104779,
-3.81401782750434));
#457312=CARTESIAN_POINT('Ctrl Pts',(-2.95767928188803,7.6719420268828,-2.44893593904025));
#457313=CARTESIAN_POINT('Ctrl Pts',(-3.66476321850187,7.83020905271775,
1.1449895334972));
#457314=CARTESIAN_POINT('Ctrl Pts',(-1.03746888674534,7.98847607855273,
3.69681543835056));
#457315=CARTESIAN_POINT('Ctrl Pts',(2.53427937155645,8.1467431043877,2.88452235506319));
#457316=CARTESIAN_POINT('Ctrl Pts',(3.79960149778944,8.30501013022267,-0.552788783937892));
#457317=CARTESIAN_POINT('Ctrl Pts',(1.60728801341828,8.46327715605764,-3.48703071577954));
#457318=CARTESIAN_POINT('Ctrl Pts',(-2.04774158557497,8.62154418189262,
-3.24800342938611));
#457319=CARTESIAN_POINT('Ctrl Pts',(-3.83925454563574,8.77981120772757,
-0.05321262973447));
#457320=CARTESIAN_POINT('Ctrl Pts',(-2.1369693841164,8.93807823356256,3.19000029143528));
#457321=CARTESIAN_POINT('Ctrl Pts',(1.51001406160273,9.09634525939752,3.53024027185438));
#457322=CARTESIAN_POINT('Ctrl Pts',(3.78284626436418,9.25461228523249,0.657878975735262));
#457323=CARTESIAN_POINT('Ctrl Pts',(2.61320234747722,9.41287931106747,-2.8131670900409));
#457324=CARTESIAN_POINT('Ctrl Pts',(-0.934517268612236,9.57114633690243,
-3.72416600917225));
#457325=CARTESIAN_POINT('Ctrl Pts',(-3.63180400568077,9.7294133627374,-1.24608733529705));
#457326=CARTESIAN_POINT('Ctrl Pts',(-3.02406506305954,9.88768038857237,
2.36595968014087));
#457327=CARTESIAN_POINT('Ctrl Pts',(0.335643394703413,10.0459474144073,
3.82492850692052));
#457328=CARTESIAN_POINT('Ctrl Pts',(3.38990850712089,10.2042144402423,1.80312361419755));
#457329=CARTESIAN_POINT('Ctrl Pts',(3.35927824390098,10.3624814660773,-1.85956560499302));
#457330=CARTESIAN_POINT('Ctrl Pts',(0.271626802545034,10.5207484919123,
-3.83000697279982));
#457331=CARTESIAN_POINT('Ctrl Pts',(-3.06321132332717,10.6790155177472,
-2.31505311119566));
#457332=CARTESIAN_POINT('Ctrl Pts',(-3.61045606250408,10.8372825435822,
1.30665280557312));
#457333=CARTESIAN_POINT('Ctrl Pts',(-0.872101995120261,10.9955495694172,
3.73927434655792));
#457334=CARTESIAN_POINT('Ctrl Pts',(2.65988512520687,11.1538165952521,2.76906945529497));
#457335=CARTESIAN_POINT('Ctrl Pts',(3.77131505484551,11.3120836210871,-0.72105290139894));
#457336=CARTESIAN_POINT('Ctrl Pts',(1.45076076404976,11.4703506469221,-3.55500038455815));
#457337=CARTESIAN_POINT('Ctrl Pts',(-2.19001948937017,11.6286176727571,
-3.15381501753567));
#457338=CARTESIAN_POINT('Ctrl Pts',(-3.83783118420082,11.786884698592,0.11741520539813));
#457339=CARTESIAN_POINT('Ctrl Pts',(-1.99312743757002,11.945151724427,3.28179486658758));
#457340=CARTESIAN_POINT('Ctrl Pts',(1.66536853135885,12.1034187502619,3.459665039226));
#457341=CARTESIAN_POINT('Ctrl Pts',(3.80834048885077,12.2616857760969,0.489159738362271));
#457342=CARTESIAN_POINT('Ctrl Pts',(2.48563422213058,12.4199528019319,-2.92649227617094));
#457343=CARTESIAN_POINT('Ctrl Pts',(-1.09905687047098,12.5782198277669,
-3.67896840500034));
#457344=CARTESIAN_POINT('Ctrl Pts',(-3.68358070511896,12.7364868536018,
-1.08349790789817));
#457345=CARTESIAN_POINT('Ctrl Pts',(-2.91596061441178,12.8947538794368,
2.49798082937362));
#457346=CARTESIAN_POINT('Ctrl Pts',(0.505251306385807,13.0530209052718,
3.80623904280589));
#457347=CARTESIAN_POINT('Ctrl Pts',(3.46667281147088,13.2112879311067,1.65073139463242));
#457348=CARTESIAN_POINT('Ctrl Pts',(3.27334161086357,13.3695549569417,-2.00698012699307));
#457349=CARTESIAN_POINT('Ctrl Pts',(0.101193574520564,13.5278219827767,
-3.83829316489704));
#457350=CARTESIAN_POINT('Ctrl Pts',(-3.16304295136811,13.6860890086117,
-2.17667033391095));
#457351=CARTESIAN_POINT('Ctrl Pts',(-3.54883700981142,13.8443560344466,
1.46577298694374));
#457352=CARTESIAN_POINT('Ctrl Pts',(-0.705106989009746,14.0026230602816,
3.7743289268053));
#457353=CARTESIAN_POINT('Ctrl Pts',(2.78028667201715,14.1608900861166,2.64815785108637));
#457354=CARTESIAN_POINT('Ctrl Pts',(3.73555509979697,14.3191571119515,-0.887898127934317));
#457355=CARTESIAN_POINT('Ctrl Pts',(1.29138138877944,14.4774241377865,-3.61594658340851));
#457356=CARTESIAN_POINT('Ctrl Pts',(-2.32797876264463,14.6356911636215,
-3.05339900556805));
#457357=CARTESIAN_POINT('Ctrl Pts',(-3.82882535498602,14.7939581894564,
0.287811126047398));
#457358=CARTESIAN_POINT('Ctrl Pts',(-1.84534982552105,14.9522252152914,
3.36710915021439));
#457359=CARTESIAN_POINT('Ctrl Pts',(1.81743264700028,15.1104922411264,3.38225451788678));
#457360=CARTESIAN_POINT('Ctrl Pts',(3.82631736185955,15.2687592669614,0.319479772331821));
#457361=CARTESIAN_POINT('Ctrl Pts',(2.35314883662822,15.4270262927963,-3.03404820718843));
#457362=CARTESIAN_POINT('Ctrl Pts',(-1.26140962782153,15.5852933186313,
-3.6264849003533));
#457363=CARTESIAN_POINT('Ctrl Pts',(-3.7281140141863,15.7435603444663,-0.918807404837155));
#457364=CARTESIAN_POINT('Ctrl Pts',(-2.80203657796488,15.9018273703012,
2.62514325169856));
#457365=CARTESIAN_POINT('Ctrl Pts',(0.67374445834164,16.0600943961362,3.77988873967954));
#457366=CARTESIAN_POINT('Ctrl Pts',(3.53681569126371,16.2183614219712,1.49535572158047));
#457367=CARTESIAN_POINT('Ctrl Pts',(3.18050688334997,16.3766284478062,-2.15096385528484));
#457368=CARTESIAN_POINT('Ctrl Pts',(-0.0686035803666589,16.5348954736411,
-3.8379695688805));
#457369=CARTESIAN_POINT('Ctrl Pts',(-3.25825270134793,16.6931624994761,
-2.03600447284782));
#457370=CARTESIAN_POINT('Ctrl Pts',(-3.47693117896336,16.851429525311,1.62620077958471));
#457371=CARTESIAN_POINT('Ctrl Pts',(-1.52194754166591,16.9569408758677,
3.06939099813719));
#457372=CARTESIAN_POINT('Ctrl Pts',(-0.454578479639251,17.009696551146,
3.22007180134991));
#457373=CARTESIAN_POINT('Ctrl Pts',(-2.49305876047795,6.99030344885397,
1.77778008111357));
#457374=CARTESIAN_POINT('Ctrl Pts',(-1.90377144804213,7.04305912413229,
2.60416345232695));
#457375=CARTESIAN_POINT('Ctrl Pts',(0.150776296851584,7.14857047468894,
3.6110253019962));
#457376=CARTESIAN_POINT('Ctrl Pts',(3.11565771198357,7.3068375005239,1.83839322693598));
#457377=CARTESIAN_POINT('Ctrl Pts',(3.2364564496792,7.46510452635889,-1.6089112174321));
#457378=CARTESIAN_POINT('Ctrl Pts',(0.416360707404361,7.62337155219384,
-3.59118160757021));
#457379=CARTESIAN_POINT('Ctrl Pts',(-2.78487514180233,7.78163857802882,
-2.30585542599669));
#457380=CARTESIAN_POINT('Ctrl Pts',(-3.45064728630157,7.93990560386378,
1.07809285103581));
#457381=CARTESIAN_POINT('Ctrl Pts',(-0.976854160889977,8.09817262969876,
3.48082683647892));
#457382=CARTESIAN_POINT('Ctrl Pts',(2.38621261860575,8.25643965553374,2.71599245116957));
#457383=CARTESIAN_POINT('Ctrl Pts',(3.57760756034172,8.41470668136869,-0.520491776266254));
#457384=CARTESIAN_POINT('Ctrl Pts',(1.51338127216689,8.57297370720367,-3.28329890889206));
#457385=CARTESIAN_POINT('Ctrl Pts',(-1.92810108703277,8.73124073303864,
-3.05823693135924));
#457386=CARTESIAN_POINT('Ctrl Pts',(-3.61494385570008,8.8895077588736,-0.0501036507524327));
#457387=CARTESIAN_POINT('Ctrl Pts',(-2.01211569931255,9.04777478470859,
3.00362266063187));
#457388=CARTESIAN_POINT('Ctrl Pts',(1.42179060781906,9.20604181054354,3.32398392140778));
#457389=CARTESIAN_POINT('Ctrl Pts',(3.56183126121867,9.36430883637851,0.619442012208283));
#457390=CARTESIAN_POINT('Ctrl Pts',(2.46052447354711,9.5225758622135,-2.64880615919596));
#457391=CARTESIAN_POINT('Ctrl Pts',(-0.879917551196401,9.68084288804845,
-3.50657943422061));
#457392=CARTESIAN_POINT('Ctrl Pts',(-3.41961373474617,9.83910991388344,
-1.1732839546985));
#457393=CARTESIAN_POINT('Ctrl Pts',(-2.8473822949226,9.99737693971839,2.22772710350288));
#457394=CARTESIAN_POINT('Ctrl Pts',(0.316033233266263,10.1556439655534,
3.60145482416686));
#457395=CARTESIAN_POINT('Ctrl Pts',(3.19185112201851,10.3139109913883,1.69777506355255));
#457396=CARTESIAN_POINT('Ctrl Pts',(3.16301044982312,10.4721780172233,-1.75091939805924));
#457397=CARTESIAN_POINT('Ctrl Pts',(0.255756847906782,10.6304450430583,
-3.60623657771004));
#457398=CARTESIAN_POINT('Ctrl Pts',(-2.88424141206268,10.7887120688932,
-2.17979478059074));
#457399=CARTESIAN_POINT('Ctrl Pts',(-3.39951305762222,10.9469790947282,
1.23031085198798));
#457400=CARTESIAN_POINT('Ctrl Pts',(-0.821148926524665,11.1052461205632,
3.52080505816739));
#457401=CARTESIAN_POINT('Ctrl Pts',(2.50447978271324,11.2635131463982,2.60728495452435));
#457402=CARTESIAN_POINT('Ctrl Pts',(3.5509737693533,11.4217801722331,-0.678924964355346));
#457403=CARTESIAN_POINT('Ctrl Pts',(1.36599921879469,11.5800471980681,-3.3472974100606));
#457404=CARTESIAN_POINT('Ctrl Pts',(-2.06206632117205,11.7383142239031,
-2.96955153250129));
#457405=CARTESIAN_POINT('Ctrl Pts',(-3.6136036549886,11.896581249738,0.110555153422237));
#457406=CARTESIAN_POINT('Ctrl Pts',(-1.87667780253363,12.054848275573,3.09005408409938));
#457407=CARTESIAN_POINT('Ctrl Pts',(1.56806840191293,12.213115301408,3.25753208797971));
#457408=CARTESIAN_POINT('Ctrl Pts',(3.58583597074448,12.371382327243,0.460580294854009));
#457409=CARTESIAN_POINT('Ctrl Pts',(2.34040959045628,12.5296493530779,-2.75551025511545));
#457410=CARTESIAN_POINT('Ctrl Pts',(-1.03484383068333,12.6879163789129,
-3.4640225264794));
#457411=CARTESIAN_POINT('Ctrl Pts',(-3.46836535026884,12.8461834047479,
-1.02019390958923));
#457412=CARTESIAN_POINT('Ctrl Pts',(-2.74559391184774,13.0044504305828,
2.35203483995757));
#457413=CARTESIAN_POINT('Ctrl Pts',(0.4757317036142,13.1627174564178,3.58385730291256));
#457414=CARTESIAN_POINT('Ctrl Pts',(3.26413042703685,13.3209844822528,1.55428644845155));
#457415=CARTESIAN_POINT('Ctrl Pts',(3.0820947147799,13.4792515080877,-1.88972114048365));
#457416=CARTESIAN_POINT('Ctrl Pts',(0.0952812808062532,13.6375185339227,
-3.61403864419272));
#457417=CARTESIAN_POINT('Ctrl Pts',(-2.97824031890811,13.7957855597577,
-2.04949709791984));
#457418=CARTESIAN_POINT('Ctrl Pts',(-3.34149413408443,13.9540525855927,
1.38013434379513));
#457419=CARTESIAN_POINT('Ctrl Pts',(-0.663910701213964,14.1123196114276,
3.55381155408297));
#457420=CARTESIAN_POINT('Ctrl Pts',(2.61784679880582,14.2705866372626,2.49343768143495));
#457421=CARTESIAN_POINT('Ctrl Pts',(3.51730311057144,14.4288536630976,-0.8360221610501));
#457422=CARTESIAN_POINT('Ctrl Pts',(1.21593167664287,14.5871206889325,-3.40468279163495));
#457423=CARTESIAN_POINT('Ctrl Pts',(-2.19196524330193,14.7453877147675,
-2.87500238470152));
#457424=CARTESIAN_POINT('Ctrl Pts',(-3.60512399660737,14.9036547406025,
0.270995592852758));
#457425=CARTESIAN_POINT('Ctrl Pts',(-1.73753418380856,15.0619217664374,
3.17038383085992));
#457426=CARTESIAN_POINT('Ctrl Pts',(1.71124808275365,15.2201887922724,3.18464432157728));
#457427=CARTESIAN_POINT('Ctrl Pts',(3.60276253444463,15.3784558181074,0.300813979975401));
#457428=CARTESIAN_POINT('Ctrl Pts',(2.21566474100726,15.5367228439424,-2.85678216802306));
#457429=CARTESIAN_POINT('Ctrl Pts',(-1.18771103333013,15.6949898697773,
-3.41460540125516));
#457430=CARTESIAN_POINT('Ctrl Pts',(-3.51029677473507,15.8532568956123,
-0.865125545390938));
#457431=CARTESIAN_POINT('Ctrl Pts',(-2.63832595379104,16.0115239214473,
2.47176772346279));
#457432=CARTESIAN_POINT('Ctrl Pts',(0.634380544723908,16.1697909472822,
3.55904653164168));
#457433=CARTESIAN_POINT('Ctrl Pts',(3.3301751680964,16.3280579731172,1.4079886898768));
#457434=CARTESIAN_POINT('Ctrl Pts',(2.99468391046051,16.4863249989522,-2.02529253532663));
#457435=CARTESIAN_POINT('Ctrl Pts',(-0.0645953761017088,16.6445920247872,
-3.61373395446251));
#457436=CARTESIAN_POINT('Ctrl Pts',(-3.0678873836185,16.8028590506221,-1.91704972197417));
#457437=CARTESIAN_POINT('Ctrl Pts',(-3.27378944341507,16.9611260764571,
1.53118904892018));
#457438=CARTESIAN_POINT('Ctrl Pts',(-1.43302686733732,17.0666374270137,
2.8900600357614));
#457439=CARTESIAN_POINT('Ctrl Pts',(-0.428019466376186,17.1193931022921,
3.03193722501028));
#457440=CARTESIAN_POINT('Ctrl Pts',(-2.33836210323078,7.1,1.66746714335669));
#457441=CARTESIAN_POINT('Ctrl Pts',(-1.78564062664172,7.15275567527832,
2.44257264372404));
#457442=CARTESIAN_POINT('Ctrl Pts',(0.141420484832718,7.25826702583498,
3.38695776202909));
#457443=CARTESIAN_POINT('Ctrl Pts',(2.92232820013613,7.41653405166992,1.72431918607449));
#457444=CARTESIAN_POINT('Ctrl Pts',(3.03563126175005,7.57480107750492,-1.50907675260125));
#457445=CARTESIAN_POINT('Ctrl Pts',(0.390525131177429,7.73306810333986,
-3.36834538763607));
#457446=CARTESIAN_POINT('Ctrl Pts',(-2.61207100171662,7.89133512917486,
-2.16277491295312));
#457447=CARTESIAN_POINT('Ctrl Pts',(-3.23653135410128,8.0496021550098,1.01119616857442));
#457448=CARTESIAN_POINT('Ctrl Pts',(-0.91623943503461,8.2078691808448,3.26483823460727));
#457449=CARTESIAN_POINT('Ctrl Pts',(2.23814586565504,8.36613620667974,2.54746254727596));
#457450=CARTESIAN_POINT('Ctrl Pts',(3.355613622894,8.52440323251474,-0.488194768594614));
#457451=CARTESIAN_POINT('Ctrl Pts',(1.41947453091551,8.68267025834969,-3.07956710200458));
#457452=CARTESIAN_POINT('Ctrl Pts',(-1.80846058849058,8.84093728418467,
-2.86847043333237));
#457453=CARTESIAN_POINT('Ctrl Pts',(-3.39063316576441,8.99920431001964,
-0.0469946717703988));
#457454=CARTESIAN_POINT('Ctrl Pts',(-1.88726201450869,9.1574713358546,2.81724502982847));
#457455=CARTESIAN_POINT('Ctrl Pts',(1.33356715403539,9.31573836168959,3.11772757096118));
#457456=CARTESIAN_POINT('Ctrl Pts',(3.34081625807316,9.47400538752454,0.581005048681307));
#457457=CARTESIAN_POINT('Ctrl Pts',(2.30784659961701,9.63227241335953,-2.48444522835102));
#457458=CARTESIAN_POINT('Ctrl Pts',(-0.825317833780566,9.79053943919448,
-3.28899285926896));
#457459=CARTESIAN_POINT('Ctrl Pts',(-3.20742346381156,9.94880646502946,
-1.10048057409996));
#457460=CARTESIAN_POINT('Ctrl Pts',(-2.67069952678566,10.1070734908644,
2.08949452686489));
#457461=CARTESIAN_POINT('Ctrl Pts',(0.29642307182911,10.2653405166994,3.3779811414132));
#457462=CARTESIAN_POINT('Ctrl Pts',(2.99379373691612,10.4236075425344,1.59242651290754));
#457463=CARTESIAN_POINT('Ctrl Pts',(2.96674265574526,10.5818745683693,-1.64227319112547));
#457464=CARTESIAN_POINT('Ctrl Pts',(0.239886893268533,10.7401415942043,
-3.38246618262026));
#457465=CARTESIAN_POINT('Ctrl Pts',(-2.70527150079818,10.8984086200393,
-2.04453644998582));
#457466=CARTESIAN_POINT('Ctrl Pts',(-3.18857005274037,11.0566756458742,
1.15396889840285));
#457467=CARTESIAN_POINT('Ctrl Pts',(-0.770195857929068,11.2149426717092,
3.30233576977685));
#457468=CARTESIAN_POINT('Ctrl Pts',(2.34907444021962,11.3732096975442,2.44550045375373));
#457469=CARTESIAN_POINT('Ctrl Pts',(3.33063248386109,11.5314767233792,-0.636797027311755));
#457470=CARTESIAN_POINT('Ctrl Pts',(1.28123767353962,11.6897437492141,-3.13959443556305));
#457471=CARTESIAN_POINT('Ctrl Pts',(-1.93411315297392,11.8480107750491,
-2.78528804746691));
#457472=CARTESIAN_POINT('Ctrl Pts',(-3.38937612577637,12.0062778008841,
0.103695101446341));
#457473=CARTESIAN_POINT('Ctrl Pts',(-1.76022816749725,12.164544826719,2.89831330161118));
#457474=CARTESIAN_POINT('Ctrl Pts',(1.470768272467,12.322811852554,3.05539913673341));
#457475=CARTESIAN_POINT('Ctrl Pts',(3.36333145263819,12.481078878389,0.432000851345749));
#457476=CARTESIAN_POINT('Ctrl Pts',(2.19518495878197,12.6393459042239,-2.58452823405996));
#457477=CARTESIAN_POINT('Ctrl Pts',(-0.970630790895669,12.7976129300589,
-3.24907664795847));
#457478=CARTESIAN_POINT('Ctrl Pts',(-3.25314999541872,12.9558799558939,
-0.956889911280283));
#457479=CARTESIAN_POINT('Ctrl Pts',(-2.5752272092837,13.1141469817289,2.20608885054153));
#457480=CARTESIAN_POINT('Ctrl Pts',(0.446212100842591,13.2724140075638,
3.36147556301922));
#457481=CARTESIAN_POINT('Ctrl Pts',(3.06158804260283,13.4306810333988,1.45784150227068));
#457482=CARTESIAN_POINT('Ctrl Pts',(2.89084781869623,13.5889480592338,-1.77246215397422));
#457483=CARTESIAN_POINT('Ctrl Pts',(0.0893689870919405,13.7472150850687,
-3.3897841234884));
#457484=CARTESIAN_POINT('Ctrl Pts',(-2.7934376864481,13.9054821109037,-1.92232386192872));
#457485=CARTESIAN_POINT('Ctrl Pts',(-3.13415125835744,14.0637491367387,
1.29449570064652));
#457486=CARTESIAN_POINT('Ctrl Pts',(-0.622714413418182,14.2220161625736,
3.33329418136064));
#457487=CARTESIAN_POINT('Ctrl Pts',(2.4554069255945,14.3802831884086,2.33871751178352));
#457488=CARTESIAN_POINT('Ctrl Pts',(3.29905112134591,14.5385502142436,-0.784146194165878));
#457489=CARTESIAN_POINT('Ctrl Pts',(1.1404819645063,14.6968172400786,-3.19341899986139));
#457490=CARTESIAN_POINT('Ctrl Pts',(-2.05595172395924,14.8550842659135,
-2.696605763835));
#457491=CARTESIAN_POINT('Ctrl Pts',(-3.38142263822873,15.0133512917485,
0.254180059658117));
#457492=CARTESIAN_POINT('Ctrl Pts',(-1.62971854209606,15.1716183175835,
2.97365851150546));
#457493=CARTESIAN_POINT('Ctrl Pts',(1.60506351850703,15.3298853434185,2.98703412526777));
#457494=CARTESIAN_POINT('Ctrl Pts',(3.37920770702971,15.4881523692534,0.282148187618979));
#457495=CARTESIAN_POINT('Ctrl Pts',(2.07818064538629,15.6464193950884,-2.67951612885769));
#457496=CARTESIAN_POINT('Ctrl Pts',(-1.11401243883872,15.8046864209233,
-3.20272590215703));
#457497=CARTESIAN_POINT('Ctrl Pts',(-3.29247953528384,15.9629534467583,
-0.811443685944723));
#457498=CARTESIAN_POINT('Ctrl Pts',(-2.47461532961719,16.1212204725933,
2.31839219522703));
#457499=CARTESIAN_POINT('Ctrl Pts',(0.595016631106169,16.2794874984283,
3.33820432360382));
#457500=CARTESIAN_POINT('Ctrl Pts',(3.12353464492909,16.4377545242632,1.32062165817314));
#457501=CARTESIAN_POINT('Ctrl Pts',(2.80886093757105,16.5960215500982,-1.89962121536842));
#457502=CARTESIAN_POINT('Ctrl Pts',(-0.0605871718367519,16.7542885759332,
-3.38949834004452));
#457503=CARTESIAN_POINT('Ctrl Pts',(-2.87752206588908,16.9125556017681,
-1.79809497110052));
#457504=CARTESIAN_POINT('Ctrl Pts',(-3.07064770786678,17.0708226276031,
1.43617731825564));
#457505=CARTESIAN_POINT('Ctrl Pts',(-1.34410619300874,17.1763339781598,
2.71072907338562));
#457506=CARTESIAN_POINT('Ctrl Pts',(-0.401460453113122,17.2290896534381,
2.84380264867065));
#457507=CARTESIAN_POINT('Ctrl Pts',(3.09699338763788,7.1,1.51441171489139));
#457508=CARTESIAN_POINT('Ctrl Pts',(3.05138631168995,7.1,1.59235606784553));
#457509=CARTESIAN_POINT('Ctrl Pts',(3.00262634822843,7.1,1.66819495986494));
#457510=CARTESIAN_POINT('Ctrl Pts',(2.9507154613905,7.1,1.74171658295999));
#457511=CARTESIAN_POINT('Ctrl Pts',(2.88808245753381,7.1,1.83042398873481));
#457512=CARTESIAN_POINT('Ctrl Pts',(2.82086319276517,7.1,1.91575934092478));
#457513=CARTESIAN_POINT('Ctrl Pts',(2.74945446377628,7.1,1.99757097072423));
#457514=CARTESIAN_POINT('Ctrl Pts',(2.67683632715039,7.1,2.08076819597225));
#457515=CARTESIAN_POINT('Ctrl Pts',(2.59988479291176,7.1,2.16032181447893));
#457516=CARTESIAN_POINT('Ctrl Pts',(2.51898429832516,7.1,2.23603014307834));
#457517=CARTESIAN_POINT('Ctrl Pts',(2.43933674623876,7.1,2.31056594259736));
#457518=CARTESIAN_POINT('Ctrl Pts',(2.35586069002669,7.1,2.38137487814425));
#457519=CARTESIAN_POINT('Ctrl Pts',(2.26890461941283,7.1,2.4482188967034));
#457520=CARTESIAN_POINT('Ctrl Pts',(2.25410139539327,7.1,2.45959828602163));
#457521=CARTESIAN_POINT('Ctrl Pts',(2.2391972920332,7.1,2.47086265479881));
#457522=CARTESIAN_POINT('Ctrl Pts',(2.22419400368059,7.1,2.48201068638687));
#457523=CARTESIAN_POINT('Ctrl Pts',(2.21171926433338,7.1,2.49127990690887));
#457524=CARTESIAN_POINT('Ctrl Pts',(2.19918335459787,7.1,2.50046318838471));
#457525=CARTESIAN_POINT('Ctrl Pts',(2.18658917112344,7.1,2.50955885869257));
#457526=CARTESIAN_POINT('Ctrl Pts',(2.09831122456602,7.1,2.5733142501375));
#457527=CARTESIAN_POINT('Ctrl Pts',(2.00714475761466,7.1,2.63278941917963));
#457528=CARTESIAN_POINT('Ctrl Pts',(1.91347510734792,7.1,2.68782542766927));
#457529=CARTESIAN_POINT('Ctrl Pts',(1.81995369108995,7.1,2.7427743406254));
#457530=CARTESIAN_POINT('Ctrl Pts',(1.72393609567924,7.1,2.79329845475051));
#457531=CARTESIAN_POINT('Ctrl Pts',(1.62578530520389,7.1,2.83919217540819));
#457532=CARTESIAN_POINT('Ctrl Pts',(1.52912370021484,7.1,2.88438957704099));
#457533=CARTESIAN_POINT('Ctrl Pts',(1.43039228956228,7.1,2.92509621946273));
#457534=CARTESIAN_POINT('Ctrl Pts',(1.32993096063056,7.1,2.96106607137733));
#457535=CARTESIAN_POINT('Ctrl Pts',(1.28191903464677,7.1,2.97825658524108));
#457536=CARTESIAN_POINT('Ctrl Pts',(1.23351196898821,7.1,2.99436445226978));
#457537=CARTESIAN_POINT('Ctrl Pts',(1.18474714873503,7.1,3.00935852034605));
#457538=CARTESIAN_POINT('Ctrl Pts',(1.15216287588125,7.1,3.01937743978118));
#457539=CARTESIAN_POINT('Ctrl Pts',(1.11941887866099,7.1,3.02889901118082));
#457540=CARTESIAN_POINT('Ctrl Pts',(1.08652644784596,7.1,3.03791321314893));
#457541=CARTESIAN_POINT('Ctrl Pts',(1.07176586969083,7.1,3.04195836363977));
#457542=CARTESIAN_POINT('Ctrl Pts',(1.05698038570037,7.1,3.04589992835325));
#457543=CARTESIAN_POINT('Ctrl Pts',(1.04217875085674,7.1,3.04973529915006));
#457544=CARTESIAN_POINT('Ctrl Pts',(0.940748947441955,7.1,3.07601759229222));
#457545=CARTESIAN_POINT('Ctrl Pts',(0.838451004717897,7.1,3.09734772782833));
#457546=CARTESIAN_POINT('Ctrl Pts',(0.73561798721121,7.1,3.11354024858967));
#457547=CARTESIAN_POINT('Ctrl Pts',(0.635624197682169,7.1,3.12928569253571));
#457548=CARTESIAN_POINT('Ctrl Pts',(0.535123733143622,7.1,3.14017332852956));
#457549=CARTESIAN_POINT('Ctrl Pts',(0.434422589760872,7.1,3.14598450424585));
#457550=CARTESIAN_POINT('Ctrl Pts',(0.334674581213765,7.1,3.15174067726976));
#457551=CARTESIAN_POINT('Ctrl Pts',(0.234729022424078,7.1,3.15251618885277));
#457552=CARTESIAN_POINT('Ctrl Pts',(0.134893270904415,7.1,3.14804909926986));
#457553=CARTESIAN_POINT('Ctrl Pts',(0.0727576360140052,7.1,3.14526887832575));
#457554=CARTESIAN_POINT('Ctrl Pts',(0.0106647685361902,7.1,3.14045671729177));
#457555=CARTESIAN_POINT('Ctrl Pts',(-0.0513069284014181,7.1,3.13364847640455));
#457556=CARTESIAN_POINT('Ctrl Pts',(-0.0783570039498824,7.1,3.13067674189587));
#457557=CARTESIAN_POINT('Ctrl Pts',(-0.10538394980607,7.1,3.12732463473769));
#457558=CARTESIAN_POINT('Ctrl Pts',(-0.132381022310655,7.1,3.12359482034564));
#457559=CARTESIAN_POINT('Ctrl Pts',(-0.148018419670001,7.1,3.12143441611236));
#457560=CARTESIAN_POINT('Ctrl Pts',(-0.163637581507457,7.1,3.1191483935117));
#457561=CARTESIAN_POINT('Ctrl Pts',(-0.179232128568581,7.1,3.11673850867025));
#457562=CARTESIAN_POINT('Ctrl Pts',(-0.278819614987809,7.1,3.10134887452577));
#457563=CARTESIAN_POINT('Ctrl Pts',(-0.377472084912431,7.1,3.08090281406002));
#457564=CARTESIAN_POINT('Ctrl Pts',(-0.474882184244777,7.1,3.05564016293009));
#457565=CARTESIAN_POINT('Ctrl Pts',(-0.574147134205758,7.1,3.02989646882155));
#457566=CARTESIAN_POINT('Ctrl Pts',(-0.672122792687237,7.1,2.99915057478039));
#457567=CARTESIAN_POINT('Ctrl Pts',(-0.76846447382552,7.1,2.96360641162069));
#457568=CARTESIAN_POINT('Ctrl Pts',(-0.864056331237232,7.1,2.9283388873629));
#457569=CARTESIAN_POINT('Ctrl Pts',(-0.958040274144051,7.1,2.88834687741555));
#457570=CARTESIAN_POINT('Ctrl Pts',(-1.05004898277166,7.1,2.8437891483571));
#457571=CARTESIAN_POINT('Ctrl Pts',(-1.09079293778152,7.1,2.82405777580358));
#457572=CARTESIAN_POINT('Ctrl Pts',(-1.13114908788126,7.1,2.8034306057743));
#457573=CARTESIAN_POINT('Ctrl Pts',(-1.17108303261526,7.1,2.78191933314891));
#457574=CARTESIAN_POINT('Ctrl Pts',(-1.19552288845622,7.1,2.76875428257797));
#457575=CARTESIAN_POINT('Ctrl Pts',(-1.21980457394424,7.1,2.7552580655895));
#457576=CARTESIAN_POINT('Ctrl Pts',(-1.24391987476384,7.1,2.74143315798034));
#457577=CARTESIAN_POINT('Ctrl Pts',(-1.25788504493234,7.1,2.73342715429123));
#457578=CARTESIAN_POINT('Ctrl Pts',(-1.27179184625963,7.1,2.72531232938243));
#457579=CARTESIAN_POINT('Ctrl Pts',(-1.28562993894826,7.1,2.71709465128527));
#457580=CARTESIAN_POINT('Ctrl Pts',(-1.372340524926,7.1,2.66560202876751));
#457581=CARTESIAN_POINT('Ctrl Pts',(-1.45645830167012,7.1,2.61001589207157));
#457582=CARTESIAN_POINT('Ctrl Pts',(-1.53764003195818,7.1,2.55051510841358));
#457583=CARTESIAN_POINT('Ctrl Pts',(-1.61843699822156,7.1,2.49129633107538));
#457584=CARTESIAN_POINT('Ctrl Pts',(-1.69632636725415,7.1,2.4281993445793));
#457585=CARTESIAN_POINT('Ctrl Pts',(-1.77092888084013,7.1,2.36136796463788));
#457586=CARTESIAN_POINT('Ctrl Pts',(-1.79272875583386,7.1,2.34183892120018));
#457587=CARTESIAN_POINT('Ctrl Pts',(-1.81424766634448,7.1,2.32199082074022));
#457588=CARTESIAN_POINT('Ctrl Pts',(-1.83547535662103,7.1,2.30182683287202));
#457589=CARTESIAN_POINT('Ctrl Pts',(-1.84945973062044,7.1,2.28854320455472));
#457590=CARTESIAN_POINT('Ctrl Pts',(-1.86331923229643,7.1,2.27512097363059));
#457591=CARTESIAN_POINT('Ctrl Pts',(-1.8770459964819,7.1,2.26156579733141));
#457592=CARTESIAN_POINT('Ctrl Pts',(-1.94633415556125,7.1,2.19314375706934));
#457593=CARTESIAN_POINT('Ctrl Pts',(-2.01210277297389,7.1,2.12147745509268));
#457594=CARTESIAN_POINT('Ctrl Pts',(-2.07401739382647,7.1,2.04671449447803));
#457595=CARTESIAN_POINT('Ctrl Pts',(-2.13419826203252,7.1,1.97404506975267));
#457596=CARTESIAN_POINT('Ctrl Pts',(-2.19073831622834,7.1,1.89844941478769));
#457597=CARTESIAN_POINT('Ctrl Pts',(-2.24328693920311,7.1,1.8200412855861));
#457598=CARTESIAN_POINT('Ctrl Pts',(-2.27661878753152,7.1,1.77030662609718));
#457599=CARTESIAN_POINT('Ctrl Pts',(-2.30834382556741,7.1,1.71943998109422));
#457600=CARTESIAN_POINT('Ctrl Pts',(-2.33836210323078,7.1,1.66746714335669));
#457601=CARTESIAN_POINT('',(-0.481137492902315,16.9,3.40820637768954));
#457602=CARTESIAN_POINT('Ctrl Pts',(-0.481137492902315,16.9,3.40820637768954));
#457603=CARTESIAN_POINT('Ctrl Pts',(-1.61086821599449,16.8472443247217,
3.24872196051297));
#457604=CARTESIAN_POINT('Ctrl Pts',(-2.64547056525308,16.7944886494434,
2.4849672353811));
#457605=CARTESIAN_POINT('Ctrl Pts',(-3.12419592397665,16.741732974165,1.45706125048672));
#457606=CARTESIAN_POINT('Ctrl Pts',(-3.60292128270023,16.6889772988867,
0.429155265592336));
#457607=CARTESIAN_POINT('Ctrl Pts',(-3.52576965088879,16.6362216236084,
-0.862901979064563));
#457608=CARTESIAN_POINT('Ctrl Pts',(-2.92452612924211,16.5834659483301,
-1.82680492798919));
#457609=CARTESIAN_POINT('Ctrl Pts',(-2.32328260759544,16.5307102730517,
-2.79070787691381));
#457610=CARTESIAN_POINT('Ctrl Pts',(-1.19794719611352,16.4779545977734,
-3.42645653010615));
#457611=CARTESIAN_POINT('Ctrl Pts',(-0.062122550227398,16.4251989224951,
-3.44673585535974));
#457612=CARTESIAN_POINT('Ctrl Pts',(-0.0414648377584936,16.4242394332157,
-3.44710468383311));
#457613=CARTESIAN_POINT('Ctrl Pts',(-0.0208036556395614,16.4232799439363,
-3.44726992612577));
#457614=CARTESIAN_POINT('Ctrl Pts',(-0.000142136989979558,16.4223204546569,
-3.44723320560186));
#457615=CARTESIAN_POINT('Ctrl Pts',(-2.95083879450908,16.9,-0.516457884956439));
#457616=CARTESIAN_POINT('Ctrl Pts',(-2.97665665724874,16.9,-0.418641055033343));
#457617=CARTESIAN_POINT('Ctrl Pts',(-2.99771031524562,16.9,-0.319615847049016));
#457618=CARTESIAN_POINT('Ctrl Pts',(-3.01401797859282,16.9,-0.219802864251303));
#457619=CARTESIAN_POINT('Ctrl Pts',(-3.03050300001566,16.9,-0.118904340369248));
#457620=CARTESIAN_POINT('Ctrl Pts',(-3.04213854325016,16.9,-0.01719992756052));
#457621=CARTESIAN_POINT('Ctrl Pts',(-3.04889618900187,16.9,0.0849005471415487));
#457622=CARTESIAN_POINT('Ctrl Pts',(-3.05595054381229,16.9,0.191483964107199));
#457623=CARTESIAN_POINT('Ctrl Pts',(-3.05768994941762,16.9,0.298500029301654));
#457624=CARTESIAN_POINT('Ctrl Pts',(-3.0540226994191,16.9,0.405494501672288));
#457625=CARTESIAN_POINT('Ctrl Pts',(-3.05352154435089,16.9,0.420116036097146));
#457626=CARTESIAN_POINT('Ctrl Pts',(-3.05291931902786,16.9,0.43473565270573));
#457627=CARTESIAN_POINT('Ctrl Pts',(-3.05221650494449,16.9,0.449340169749314));
#457628=CARTESIAN_POINT('Ctrl Pts',(-3.04717082651286,16.9,0.554189657535853));
#457629=CARTESIAN_POINT('Ctrl Pts',(-3.03693930777746,16.9,0.658428042447195));
#457630=CARTESIAN_POINT('Ctrl Pts',(-3.0215319722778,16.9,0.761619901782156));
#457631=CARTESIAN_POINT('Ctrl Pts',(-3.00620861576567,16.9,0.864249305144831));
#457632=CARTESIAN_POINT('Ctrl Pts',(-2.9857658698597,16.9,0.965844543239253));
#457633=CARTESIAN_POINT('Ctrl Pts',(-2.96016437649631,16.9,1.06598987532431));
#457634=CARTESIAN_POINT('Ctrl Pts',(-2.93637971082258,16.9,1.15902832462952));
#457635=CARTESIAN_POINT('Ctrl Pts',(-2.90814215886226,16.9,1.25081609535364));
#457636=CARTESIAN_POINT('Ctrl Pts',(-2.87537983234519,16.9,1.34101850078862));
#457637=CARTESIAN_POINT('Ctrl Pts',(-2.85211250745606,16.9,1.40507892921831));
#457638=CARTESIAN_POINT('Ctrl Pts',(-2.82656219568971,16.9,1.4683397228178));
#457639=CARTESIAN_POINT('Ctrl Pts',(-2.79881563558833,16.9,1.53074168394433));
#457640=CARTESIAN_POINT('Ctrl Pts',(-2.79101207619887,16.9,1.54829187423423));
#457641=CARTESIAN_POINT('Ctrl Pts',(-2.78303473738331,16.9,1.56577411033552));
#457642=CARTESIAN_POINT('Ctrl Pts',(-2.77488541132478,16.9,1.58318701982711));
#457643=CARTESIAN_POINT('Ctrl Pts',(-2.76883812508864,16.9,1.59610843776319));
#457644=CARTESIAN_POINT('Ctrl Pts',(-2.76269766084434,16.9,1.6089883219928));
#457645=CARTESIAN_POINT('Ctrl Pts',(-2.75646860826711,16.9,1.62181874485785));
#457646=CARTESIAN_POINT('Ctrl Pts',(-2.71214573987275,16.9,1.71311371099289));
#457647=CARTESIAN_POINT('Ctrl Pts',(-2.66328947658821,16.9,1.80201746569949));
#457648=CARTESIAN_POINT('Ctrl Pts',(-2.61026832672044,16.9,1.88836191237357));
#457649=CARTESIAN_POINT('Ctrl Pts',(-2.55591587729441,16.9,1.97687436792717));
#457650=CARTESIAN_POINT('Ctrl Pts',(-2.4971864760472,16.9,2.06269796096898));
#457651=CARTESIAN_POINT('Ctrl Pts',(-2.43442373776504,16.9,2.14564097133398));
#457652=CARTESIAN_POINT('Ctrl Pts',(-2.3703172711337,16.9,2.23035976263915));
#457653=CARTESIAN_POINT('Ctrl Pts',(-2.30200252139198,16.9,2.31207399252615));
#457654=CARTESIAN_POINT('Ctrl Pts',(-2.22979594959464,16.9,2.39055866186983));
#457655=CARTESIAN_POINT('Ctrl Pts',(-2.17205037665802,16.9,2.45332500134807));
#457656=CARTESIAN_POINT('Ctrl Pts',(-2.11181465263588,16.9,2.514025560767));
#457657=CARTESIAN_POINT('Ctrl Pts',(-2.04923130743126,16.9,2.57253148290693));
#457658=CARTESIAN_POINT('Ctrl Pts',(-2.03367601033663,16.9,2.58707332303559));
#457659=CARTESIAN_POINT('Ctrl Pts',(-2.01797313835135,16.9,2.6014815998716));
#457660=CARTESIAN_POINT('Ctrl Pts',(-2.00214415374043,16.9,2.61573711032485));
#457661=CARTESIAN_POINT('Ctrl Pts',(-1.92090172313698,16.9,2.68890366820473));
#457662=CARTESIAN_POINT('Ctrl Pts',(-1.83624321763956,16.9,2.75814154583534));
#457663=CARTESIAN_POINT('Ctrl Pts',(-1.74852417421841,16.9,2.82322932329071));
#457664=CARTESIAN_POINT('Ctrl Pts',(-1.66023056131919,16.9,2.88874343291823));
#457665=CARTESIAN_POINT('Ctrl Pts',(-1.56883558826159,16.9,2.95005359433295));
#457666=CARTESIAN_POINT('Ctrl Pts',(-1.4746593948356,16.9,3.00690315349514));
#457667=CARTESIAN_POINT('Ctrl Pts',(-1.43136482290328,16.9,3.03303796781425));
#457668=CARTESIAN_POINT('Ctrl Pts',(-1.38748193232619,16.9,3.05822958055756));
#457669=CARTESIAN_POINT('Ctrl Pts',(-1.34303938800765,16.9,3.08245025734981));
#457670=CARTESIAN_POINT('Ctrl Pts',(-1.32209356895734,16.9,3.09386548843402));
#457671=CARTESIAN_POINT('Ctrl Pts',(-1.30102083757109,16.9,3.10506623219387));
#457672=CARTESIAN_POINT('Ctrl Pts',(-1.27984620853268,16.9,3.11603835315651));
#457673=CARTESIAN_POINT('Ctrl Pts',(-1.18059898650193,16.9,3.1674655835156));
#457674=CARTESIAN_POINT('Ctrl Pts',(-1.07901924295251,16.9,3.2139275868326));
#457675=CARTESIAN_POINT('Ctrl Pts',(-0.975447865270529,16.9,3.25517602269448));
#457676=CARTESIAN_POINT('Ctrl Pts',(-0.873362763874905,16.9,3.29583253274208));
#457677=CARTESIAN_POINT('Ctrl Pts',(-0.769342057532994,16.9,3.3314245874836));
#457678=CARTESIAN_POINT('Ctrl Pts',(-0.663681668072933,16.9,3.36167482802888));
#457679=CARTESIAN_POINT('Ctrl Pts',(-0.603351390250923,16.9,3.37894719874042));
#457680=CARTESIAN_POINT('Ctrl Pts',(-0.54248603792155,16.9,3.39447725268593));
#457681=CARTESIAN_POINT('Ctrl Pts',(-0.481137492902315,16.9,3.40820637768954));
#457682=CARTESIAN_POINT('Origin',(0.,21.9,0.));
#457683=CARTESIAN_POINT('',(3.67394039744206E-16,21.4,-3.));
#457684=CARTESIAN_POINT('',(-3.67394039744206E-16,21.4,3.));
#457685=CARTESIAN_POINT('Origin',(0.,21.4,0.));
#457686=CARTESIAN_POINT('Origin',(0.,21.4,0.));
#457687=CARTESIAN_POINT('',(-3.06161699786838E-16,21.9,2.5));
#457688=CARTESIAN_POINT('',(-3.06161699786838E-16,21.9,2.5));
#457689=CARTESIAN_POINT('Origin',(0.,21.9,0.));
#457690=CARTESIAN_POINT('Origin',(0.,0.,0.));
#457691=CARTESIAN_POINT('',(-1.71450551880629E-16,7.1,-1.4));
#457692=CARTESIAN_POINT('Origin',(0.,7.1,0.));
#457693=CARTESIAN_POINT('',(-1.71450551880629E-16,0.,-1.4));
#457694=CARTESIAN_POINT('Origin',(0.,0.,0.));
#457695=CARTESIAN_POINT('Origin',(0.,16.9,0.));
#457696=CARTESIAN_POINT('Origin',(0.,0.,0.));
#457697=CARTESIAN_POINT('',(-3.67394039744206E-16,0.,-3.));
#457698=CARTESIAN_POINT('Origin',(0.,16.9,0.));
#457699=CARTESIAN_POINT('Origin',(0.,0.,0.));
#457700=CARTESIAN_POINT('',(-2.57175827820944E-16,16.9,-2.1));
#457701=CARTESIAN_POINT('Origin',(0.,16.9,0.));
#457702=CARTESIAN_POINT('',(-2.57175827820944E-16,21.9,-2.1));
#457703=CARTESIAN_POINT('',(-2.57175827820944E-16,0.,-2.1));
#457704=CARTESIAN_POINT('Origin',(0.,21.9,0.));
#457705=CARTESIAN_POINT('Origin',(0.,16.9,0.));
#457706=CARTESIAN_POINT('',(-1.22464679914735E-16,15.8,-0.999999999999999));
#457707=CARTESIAN_POINT('Origin',(0.,15.8,0.));
#457708=CARTESIAN_POINT('',(-2.57175827820944E-16,16.9,-2.1));
#457709=CARTESIAN_POINT('Origin',(0.,0.,0.));
#457710=CARTESIAN_POINT('',(-1.22464679914735E-16,0.,-1.));
#457711=CARTESIAN_POINT('Origin',(0.,0.,0.));
#457712=CARTESIAN_POINT('',(-1.22464679914735E-16,0.,-1.));
#457713=CARTESIAN_POINT('Origin',(2.1,21.9,0.));
#457714=CARTESIAN_POINT('Origin',(3.5,16.9,0.));
#457715=CARTESIAN_POINT('Origin',(1.4,7.1,0.));
#457716=CARTESIAN_POINT('Origin',(1.,0.,0.));
#459212=UNCERTAINTY_MEASURE_WITH_UNIT(LENGTH_MEASURE(0.01),#459243,
'DISTANCE_ACCURACY_VALUE',
'Maximum model space distance between geometric entities at asserted c
onnectivities');
#459216=UNCERTAINTY_MEASURE_WITH_UNIT(LENGTH_MEASURE(0.01),#459243,
'DISTANCE_ACCURACY_VALUE',
'Maximum model space distance between geometric entities at asserted c
onnectivities');
#459238=(
GEOMETRIC_REPRESENTATION_CONTEXT(3)
GLOBAL_UNCERTAINTY_ASSIGNED_CONTEXT((#459212))
GLOBAL_UNIT_ASSIGNED_CONTEXT((#459243,#459245,#459246))
REPRESENTATION_CONTEXT('','3D')
);
#459242=(
GEOMETRIC_REPRESENTATION_CONTEXT(3)
GLOBAL_UNCERTAINTY_ASSIGNED_CONTEXT((#459216))
GLOBAL_UNIT_ASSIGNED_CONTEXT((#459243,#459245,#459246))
REPRESENTATION_CONTEXT('','3D')
);
#459243=(
LENGTH_UNIT()
NAMED_UNIT(*)
SI_UNIT(.MILLI.,.METRE.)
);
#459245=(
NAMED_UNIT(*)
PLANE_ANGLE_UNIT()
SI_UNIT($,.RADIAN.)
);
#459246=(
NAMED_UNIT(*)
SI_UNIT($,.STERADIAN.)
SOLID_ANGLE_UNIT()
);
#459268=SHAPE_DEFINITION_REPRESENTATION(#459295,#459349);
#459295=PRODUCT_DEFINITION_SHAPE('',$,#459375);
#459349=SHAPE_REPRESENTATION('',(#105363),#459238);
#459353=PRODUCT_DEFINITION_CONTEXT('part definition',#459430,'design');
#459375=PRODUCT_DEFINITION('Hotend Heatbreak','Hotend Heatbreak',#459400,
#459353);
#459400=PRODUCT_DEFINITION_FORMATION('',$,#459453);
#459430=APPLICATION_CONTEXT(
'Core Data for Automotive Mechanical Design Process');
#459431=PRODUCT_CONTEXT('part definition',#459430,'mechanical');
#459453=PRODUCT('Hotend Heatbreak','Hotend Heatbreak',$,(#459431));
#459513=COLOUR_RGB('Sky Blue',0.24,0.69,0.87);
#459514=FILL_AREA_STYLE_COLOUR('',#459513);
#459515=FILL_AREA_STYLE('',(#459514));
#459516=SURFACE_STYLE_FILL_AREA(#459515);
#459517=SURFACE_SIDE_STYLE('',(#459516));
#459518=SURFACE_STYLE_USAGE(.BOTH.,#459517);
#459519=PRESENTATION_STYLE_ASSIGNMENT((#459518));
ENDSEC;
END-ISO-10303-21;
